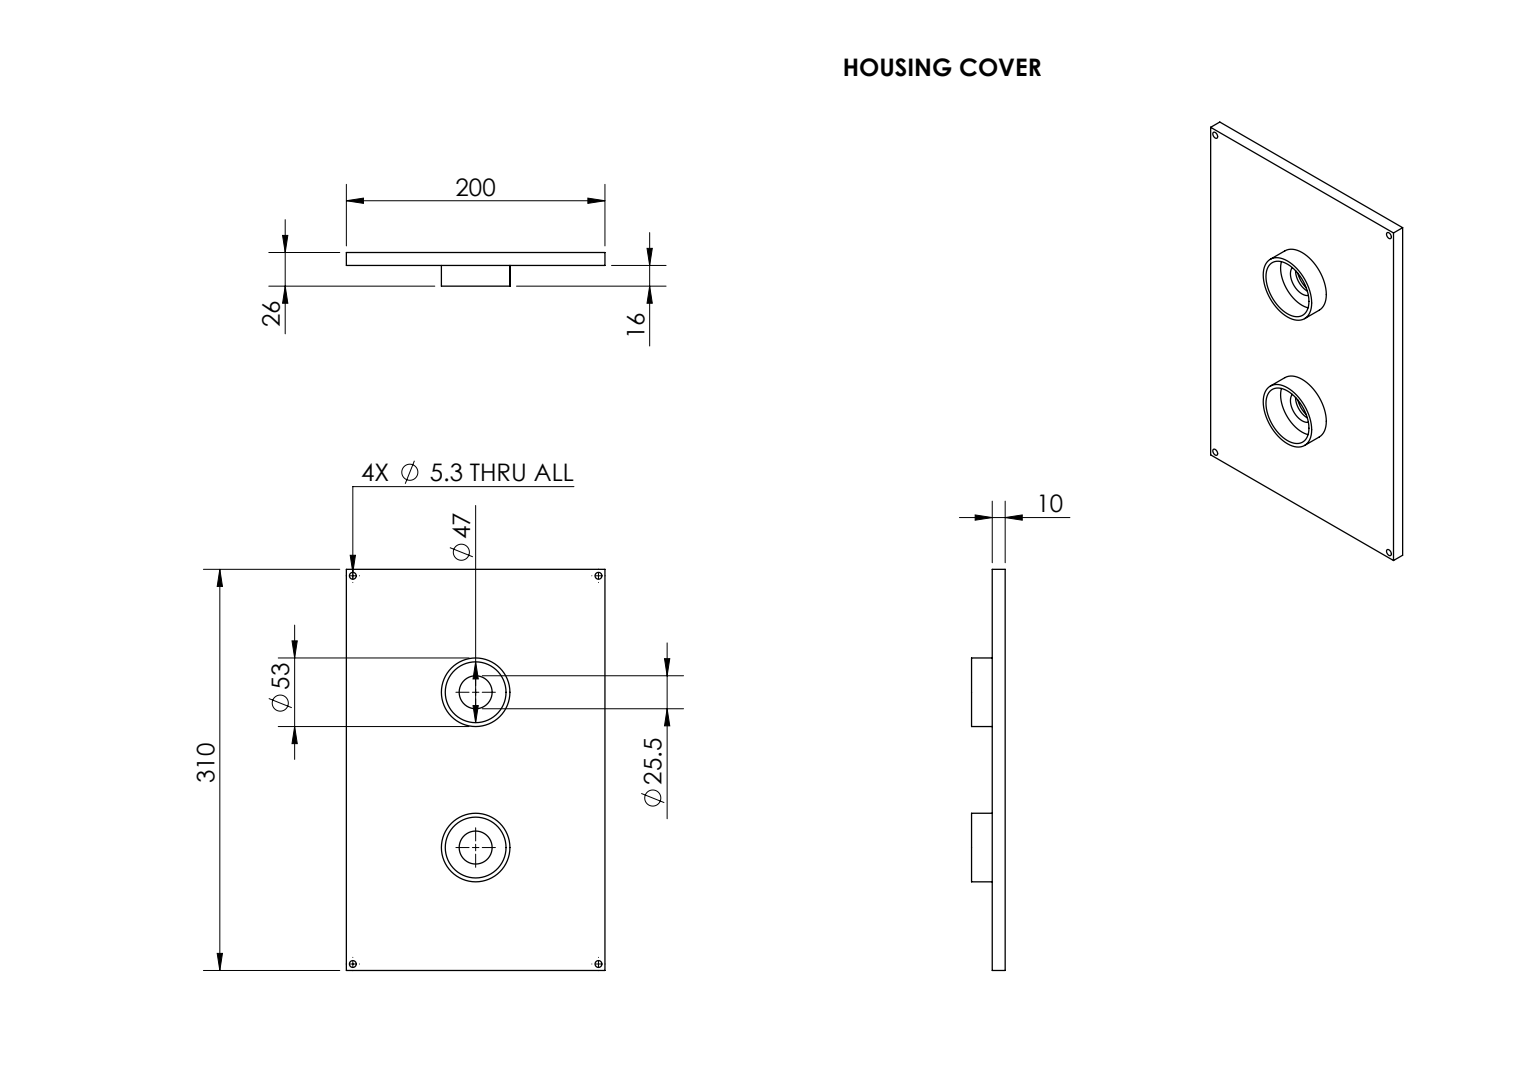
ISO-10303-21;
HEADER;
FILE_DESCRIPTION (('STEP AP214'),
    '1' );
FILE_NAME ('housing cover.step',
    '2026-10-08T09:53:37',
    ( '' ),
    ( '' ),
    'SwSTEP 2.0',
    'SolidWorks 2026',
    '' );
FILE_SCHEMA (( 'AUTOMOTIVE_DESIGN' ));
ENDSEC;

DATA;
#75=VERTEX_POINT ( 'NONE', #9336 ) ;
#149=ORIENTED_EDGE ( 'NONE', *, *, #29009, .F. ) ;
#225=AXIS2_PLACEMENT_3D ( 'NONE', #13248, #59124, #26003 ) ;
#235=EDGE_CURVE ( 'NONE', #35660, #27140, #36937, .T. ) ;
#309=CARTESIAN_POINT ( 'NONE',  ( -100.0000000000260485, 95.00000000000001421, -75.00000000000000000 ) ) ;
#339=DIRECTION ( 'NONE',  ( -1.000000000000000000, 7.571537405616606460E-15, 2.598394312951952234E-14 ) ) ;
#353=ORIENTED_EDGE ( 'NONE', *, *, #72482, .T. ) ;
#452=CYLINDRICAL_SURFACE ( 'NONE', #60264, 2.650000000000540812 ) ;
#531=LINE ( 'NONE', #23425, #23947 ) ;
#665=VECTOR ( 'NONE', #62386, 1000.000000000000000 ) ;
#686=ORIENTED_EDGE ( 'NONE', *, *, #12634, .T. ) ;
#690=CARTESIAN_POINT ( 'NONE',  ( 23.50000000000218847, -119.9999999999999716, -48.99999999999936051 ) ) ;
#767=AXIS2_PLACEMENT_3D ( 'NONE', #73077, #44536, #67455 ) ;
#820=DIRECTION ( 'NONE',  ( -2.603472992746261562E-14, -2.546204323184492723E-14, 1.000000000000000000 ) ) ;
#840=CARTESIAN_POINT ( 'NONE',  ( -0.0004442498512760095037, 0.001194404164628348752, -49.00000000000000000 ) ) ;
#873=LINE ( 'NONE', #58714, #8919 ) ;
#960=ORIENTED_EDGE ( 'NONE', *, *, #66954, .T. ) ;
#1095=VECTOR ( 'NONE', #67288, 1000.000000000000000 ) ;
#1388=DIRECTION ( 'NONE',  ( -1.000000000000000000, 7.955419762439749020E-15, 2.563413034563919251E-14 ) ) ;
#1416=ADVANCED_FACE ( 'NONE', ( #10037 ), #32956, .F. ) ;
#1664=FACE_OUTER_BOUND ( 'NONE', #62733, .T. ) ;
#1775=CIRCLE ( 'NONE', #40207, 12.75000000000265565 ) ;
#1848=CARTESIAN_POINT ( 'NONE',  ( 95.00000000002596323, -209.9999999999999147, -64.99999999999349143 ) ) ;
#1879=CIRCLE ( 'NONE', #16226, 26.50000000000552092 ) ;
#2199=CYLINDRICAL_SURFACE ( 'NONE', #34816, 2.650000000000540812 ) ;
#2442=ADVANCED_FACE ( 'NONE', ( #59711 ), #30006, .F. ) ;
#2449=AXIS2_PLACEMENT_3D ( 'NONE', #19349, #59212, #6604 ) ;
#2456=VERTEX_POINT ( 'NONE', #70970 ) ;
#2468=DIRECTION ( 'NONE',  ( 1.000000000000000000, -7.571539615859142926E-15, -2.592266024478009537E-14 ) ) ;
#2785=CARTESIAN_POINT ( 'NONE',  ( -100.0000000000260485, 95.00000000000001421, 75.00000000000001421 ) ) ;
#2842=ORIENTED_EDGE ( 'NONE', *, *, #51935, .T. ) ;
#2994=ADVANCED_FACE ( 'NONE', ( #23240 ), #21740, .F. ) ;
#3108=PLANE ( 'NONE',  #225 ) ;
#3141=DIRECTION ( 'NONE',  ( 2.603472992746261562E-14, 2.546204323184492723E-14, -1.000000000000000000 ) ) ;
#3340=DIRECTION ( 'NONE',  ( -1.000000000000000000, 7.571543891232750625E-15, 2.563413034563919882E-14 ) ) ;
#3419=VECTOR ( 'NONE', #71589, 1000.000000000000000 ) ;
#3801=FACE_OUTER_BOUND ( 'NONE', #55805, .T. ) ;
#4047=LINE ( 'NONE', #26942, #70051 ) ;
#4203=ORIENTED_EDGE ( 'NONE', *, *, #69812, .T. ) ;
#4207=ADVANCED_FACE ( 'NONE', ( #71116, #8723 ), #3108, .T. ) ;
#4229=DIRECTION ( 'NONE',  ( -1.000000000000000000, 7.677074106448950501E-15, 2.598394312951952234E-14 ) ) ;
#4446=FACE_OUTER_BOUND ( 'NONE', #31443, .T. ) ;
#4524=LINE ( 'NONE', #61285, #1095 ) ;
#4609=AXIS2_PLACEMENT_3D ( 'NONE', #43719, #49336, #66995 ) ;
#4688=CARTESIAN_POINT ( 'NONE',  ( -0.0004442498507136653329, 0.001194404164628348752, -70.59999999999999432 ) ) ;
#4779=VECTOR ( 'NONE', #23199, 1000.000000000000000 ) ;
#4855=CARTESIAN_POINT ( 'NONE',  ( -0.0004442498512760095037, 0.001194404164628348752, -49.00000000000000000 ) ) ;
#4888=DIRECTION ( 'NONE',  ( -1.000000000000000000, 5.236901059551556403E-15, 2.618450529775778123E-14 ) ) ;
#4891=DIRECTION ( 'NONE',  ( -1.000000000000000000, 1.047380211910311281E-14, 2.618450529775778123E-14 ) ) ;
#4973=VECTOR ( 'NONE', #29994, 1000.000000000000000 ) ;
#5079=COLOUR_RGB ( '', 0.66274510, 0.83137255, 0.94901961) ;
#5184=AXIS2_PLACEMENT_3D ( 'NONE', #13484, #8955, #36780 ) ;
#5204=( NAMED_UNIT ( * ) PLANE_ANGLE_UNIT ( ) SI_UNIT ( $, .RADIAN. ) );
#5224=DIRECTION ( 'NONE',  ( -1.000000000000000000, 7.571544473058805744E-15, 2.612289469705706870E-14 ) ) ;
#5225=ORIENTED_EDGE ( 'NONE', *, *, #49422, .T. ) ;
#5233=EDGE_CURVE ( 'NONE', #22100, #20743, #33218, .T. ) ;
#5362=EDGE_CURVE ( 'NONE', #75, #7432, #54715, .T. ) ;
#5427=CARTESIAN_POINT ( 'NONE',  ( -100.0000000000260059, -214.9999999999999716, 75.00000000001300293 ) ) ;
#5570=EDGE_LOOP ( 'NONE', ( #66507, #70540, #51036, #5665 ) ) ;
#5573=LINE ( 'NONE', #39398, #68174 ) ;
#5609=CARTESIAN_POINT ( 'NONE',  ( 1.692257445284848207E-12, 0.000000000000000000, -65.00000000000000000 ) ) ;
#5612=EDGE_CURVE ( 'NONE', #64620, #51781, #64388, .T. ) ;
#5619=DIRECTION ( 'NONE',  ( 2.603472992746261562E-14, 2.546204323184492723E-14, -1.000000000000000000 ) ) ;
#5665=ORIENTED_EDGE ( 'NONE', *, *, #64179, .F. ) ;
#5726=DIRECTION ( 'NONE',  ( 2.603472992746261562E-14, 2.546204323184492723E-14, -1.000000000000000000 ) ) ;
#5837=ORIENTED_EDGE ( 'NONE', *, *, #8050, .F. ) ;
#5860=ORIENTED_EDGE ( 'NONE', *, *, #50226, .F. ) ;
#5883=CYLINDRICAL_SURFACE ( 'NONE', #15596, 2.650000000000540812 ) ;
#5913=AXIS2_PLACEMENT_3D ( 'NONE', #70534, #20538, #66412 ) ;
#5943=SURFACE_STYLE_USAGE ( .BOTH. , #40137 ) ;
#5966=CARTESIAN_POINT ( 'NONE',  ( 95.00000000002596323, -209.9999999999999147, -74.99999999999349143 ) ) ;
#6234=DIRECTION ( 'NONE',  ( -1.000000000000000000, 7.571541139944061634E-15, 2.603472992745718826E-14 ) ) ;
#6399=FACE_OUTER_BOUND ( 'NONE', #37814, .T. ) ;
#6400=EDGE_CURVE ( 'NONE', #46991, #57518, #64592, .T. ) ;
#6460=DIRECTION ( 'NONE',  ( -1.000000000000000000, 1.047380211910311281E-14, 2.618450529775778123E-14 ) ) ;
#6484=EDGE_CURVE ( 'NONE', #55201, #43013, #21999, .T. ) ;
#6562=EDGE_CURVE ( 'NONE', #6768, #30711, #66814, .T. ) ;
#6604=DIRECTION ( 'NONE',  ( 1.000000000000000000, -7.331661483372147883E-15, -2.618450529775767079E-14 ) ) ;
#6633=AXIS2_PLACEMENT_3D ( 'NONE', #30357, #53302, #68759 ) ;
#6748=ORIENTED_EDGE ( 'NONE', *, *, #72073, .T. ) ;
#6768=VERTEX_POINT ( 'NONE', #22819 ) ;
#6798=EDGE_CURVE ( 'NONE', #52133, #14126, #31591, .T. ) ;
#6966=FACE_BOUND ( 'NONE', #58248, .T. ) ;
#7043=ADVANCED_FACE ( 'NONE', ( #9205 ), #20107, .F. ) ;
#7102=( NAMED_UNIT ( * ) SI_UNIT ( $, .STERADIAN. ) SOLID_ANGLE_UNIT ( ) );
#7116=VECTOR ( 'NONE', #65821, 1000.000000000000000 ) ;
#7300=ORIENTED_EDGE ( 'NONE', *, *, #67968, .T. ) ;
#7314=ORIENTED_EDGE ( 'NONE', *, *, #40834, .T. ) ;
#7352=FACE_BOUND ( 'NONE', #46868, .T. ) ;
#7414=EDGE_CURVE ( 'NONE', #49091, #67107, #23299, .T. ) ;
#7432=VERTEX_POINT ( 'NONE', #58557 ) ;
#7636=LINE ( 'NONE', #26027, #7750 ) ;
#7668=DIRECTION ( 'NONE',  ( 2.603472992746261562E-14, 2.546204323184492723E-14, -1.000000000000000000 ) ) ;
#7690=LINE ( 'NONE', #70091, #54295 ) ;
#7703=CIRCLE ( 'NONE', #34100, 2.650000000000540812 ) ;
#7750=VECTOR ( 'NONE', #71142, 1000.000000000000000 ) ;
#7840=ORIENTED_EDGE ( 'NONE', *, *, #5233, .T. ) ;
#7863=EDGE_LOOP ( 'NONE', ( #49210, #51401, #64566, #45309 ) ) ;
#7920=DIRECTION ( 'NONE',  ( 2.603472992746261562E-14, 2.546204323184492723E-14, -1.000000000000000000 ) ) ;
#8001=DIRECTION ( 'NONE',  ( 2.603472992746261562E-14, 2.546204323184492723E-14, -1.000000000000000000 ) ) ;
#8050=EDGE_CURVE ( 'NONE', #22100, #25604, #71592, .T. ) ;
#8245=CIRCLE ( 'NONE', #43094, 15.70000000000326956 ) ;
#8272=DIRECTION ( 'NONE',  ( 1.000000000000000000, 7.705842312278612278E-15, -2.603472992745757322E-14 ) ) ;
#8281=CIRCLE ( 'NONE', #46716, 2.650000000000540812 ) ;
#8322=ORIENTED_EDGE ( 'NONE', *, *, #10250, .T. ) ;
#8346=EDGE_LOOP ( 'NONE', ( #14630, #70144 ) ) ;
#8485=ADVANCED_FACE ( 'NONE', ( #1664, #40738 ), #12883, .T. ) ;
#8538=DIRECTION ( 'NONE',  ( -1.000000000000000000, 7.955419762439749020E-15, 2.563413034563919251E-14 ) ) ;
#8610=CYLINDRICAL_SURFACE ( 'NONE', #37131, 23.50000000000489919 ) ;
#8715=AXIS2_PLACEMENT_3D ( 'NONE', #4688, #74197, #50136 ) ;
#8723=FACE_OUTER_BOUND ( 'NONE', #71462, .T. ) ;
#8892=ORIENTED_EDGE ( 'NONE', *, *, #22702, .F. ) ;
#8901=CARTESIAN_POINT ( 'NONE',  ( 2.861260715122138586E-12, -120.0000000000000000, -75.00000000000000000 ) ) ;
#8906=EDGE_CURVE ( 'NONE', #42522, #22100, #70571, .T. ) ;
#8919=VECTOR ( 'NONE', #64363, 1000.000000000000000 ) ;
#8955=DIRECTION ( 'NONE',  ( -2.603472992746261562E-14, -2.546204323184492723E-14, 1.000000000000000000 ) ) ;
#8981=DIRECTION ( 'NONE',  ( 2.603472992746261562E-14, 2.546204323184492723E-14, -1.000000000000000000 ) ) ;
#9143=PRODUCT_DEFINITION_SHAPE ( 'NONE', 'NONE',  #31551 ) ;
#9205=FACE_OUTER_BOUND ( 'NONE', #18582, .T. ) ;
#9263=DIRECTION ( 'NONE',  ( -2.603472992746261562E-14, -2.546204323184492723E-14, 1.000000000000000000 ) ) ;
#9336=CARTESIAN_POINT ( 'NONE',  ( -92.35000000002612808, 89.99999999999992895, -74.99999999999992895 ) ) ;
#9493=DIRECTION ( 'NONE',  ( 2.603472992746261562E-14, 2.546204323184492723E-14, -1.000000000000000000 ) ) ;
#9614=EDGE_CURVE ( 'NONE', #64620, #52133, #33989, .T. ) ;
#9626=LINE ( 'NONE', #67136, #51555 ) ;
#9698=DIRECTION ( 'NONE',  ( 2.603472992746261562E-14, 2.546204323184492723E-14, -1.000000000000000000 ) ) ;
#9849=CYLINDRICAL_SURFACE ( 'NONE', #24494, 23.50000000000489919 ) ;
#9867=ORIENTED_EDGE ( 'NONE', *, *, #51725, .T. ) ;
#9970=DIRECTION ( 'NONE',  ( 2.603472992746261562E-14, 2.546204323184492723E-14, -1.000000000000000000 ) ) ;
#9980=ORIENTED_EDGE ( 'NONE', *, *, #42054, .T. ) ;
#10036=AXIS2_PLACEMENT_3D ( 'NONE', #43811, #31757, #55442 ) ;
#10037=FACE_OUTER_BOUND ( 'NONE', #23609, .T. ) ;
#10227=DIRECTION ( 'NONE',  ( -7.571541139946887334E-15, 1.000000000000000000, 2.546204323184473159E-14 ) ) ;
#10250=EDGE_CURVE ( 'NONE', #25604, #73822, #39518, .T. ) ;
#10297=DIRECTION ( 'NONE',  ( 2.603472992745699578E-14, -2.546204323184531851E-14, 1.000000000000000000 ) ) ;
#10346=CYLINDRICAL_SURFACE ( 'NONE', #53211, 12.75000000000265565 ) ;
#10395=VERTEX_POINT ( 'NONE', #19525 ) ;
#10400=MECHANICAL_DESIGN_GEOMETRIC_PRESENTATION_REPRESENTATION('',(#28426),#23610);
#10430=DIRECTION ( 'NONE',  ( -1.000000000000000000, 7.571539615859142926E-15, 2.592266024478009537E-14 ) ) ;
#10480=FACE_BOUND ( 'NONE', #35331, .T. ) ;
#10514=FILL_AREA_STYLE_COLOUR ( '', #18810 ) ;
#10593=CARTESIAN_POINT ( 'NONE',  ( 2.746707903440850533E-12, -120.0000000000000000, -70.59999999999999432 ) ) ;
#10809=CIRCLE ( 'NONE', #45664, 12.75000000000265565 ) ;
#10887=CARTESIAN_POINT ( 'NONE',  ( -15.70044424985387188, 0.001194404164747221980, -74.99999999999958789 ) ) ;
#10892=ADVANCED_FACE ( 'NONE', ( #42388 ), #2199, .F. ) ;
#11106=DIRECTION ( 'NONE',  ( 2.603472992746261562E-14, 2.546204323184492723E-14, -1.000000000000000000 ) ) ;
#11125=ADVANCED_FACE ( 'NONE', ( #66075 ), #5883, .F. ) ;
#11158=CARTESIAN_POINT ( 'NONE',  ( 26.49955575014914189, 0.001194404164634644498, -64.99999999999930367 ) ) ;
#11179=CARTESIAN_POINT ( 'NONE',  ( -0.0004442498512760095037, 0.001194404164628348752, -49.00000000000000000 ) ) ;
#11423=DIRECTION ( 'NONE',  ( 2.603472992746261562E-14, 2.546204323184492723E-14, -1.000000000000000000 ) ) ;
#11448=ORIENTED_EDGE ( 'NONE', *, *, #19451, .T. ) ;
#11479=ORIENTED_EDGE ( 'NONE', *, *, #70861, .T. ) ;
#11501=DIRECTION ( 'NONE',  ( 2.603472992746261562E-14, 2.546204323184492723E-14, -1.000000000000000000 ) ) ;
#11616=ORIENTED_EDGE ( 'NONE', *, *, #63442, .T. ) ;
#11629=ORIENTED_EDGE ( 'NONE', *, *, #46112, .T. ) ;
#11782=CIRCLE ( 'NONE', #34598, 15.70000000000326956 ) ;
#11845=ADVANCED_FACE ( 'NONE', ( #67637 ), #66530, .F. ) ;
#11937=ORIENTED_EDGE ( 'NONE', *, *, #9614, .F. ) ;
#12024=VECTOR ( 'NONE', #59259, 1000.000000000000000 ) ;
#12175=FACE_OUTER_BOUND ( 'NONE', #28138, .T. ) ;
#12199=ORIENTED_EDGE ( 'NONE', *, *, #45524, .T. ) ;
#12209=CARTESIAN_POINT ( 'NONE',  ( 23.50000000000260414, -119.9999999999999716, -64.99999999999938893 ) ) ;
#12296=DIRECTION ( 'NONE',  ( 2.603472992746261562E-14, 2.546204323184492723E-14, -1.000000000000000000 ) ) ;
#12317=CIRCLE ( 'NONE', #53159, 2.650000000000540812 ) ;
#12387=AXIS2_PLACEMENT_3D ( 'NONE', #1848, #48405, #30366 ) ;
#12417=VECTOR ( 'NONE', #64516, 1000.000000000000000 ) ;
#12534=DIRECTION ( 'NONE',  ( -1.000000000000000000, 7.677074106448950501E-15, 2.598394312951952234E-14 ) ) ;
#12627=LINE ( 'NONE', #35565, #12417 ) ;
#12634=EDGE_CURVE ( 'NONE', #10395, #2456, #65815, .T. ) ;
#12779=EDGE_LOOP ( 'NONE', ( #43223, #52931, #15236, #53707 ) ) ;
#12814=VECTOR ( 'NONE', #59888, 1000.000000000000000 ) ;
#12841=VECTOR ( 'NONE', #37141, 1000.000000000000000 ) ;
#12883=PLANE ( 'NONE',  #66193 ) ;
#12972=ORIENTED_EDGE ( 'NONE', *, *, #23448, .F. ) ;
#13036=ORIENTED_EDGE ( 'NONE', *, *, #8906, .T. ) ;
#13180=CIRCLE ( 'NONE', #2449, 26.50000000000552092 ) ;
#13248=CARTESIAN_POINT ( 'NONE',  ( 1.692257445284848207E-12, 0.000000000000000000, -65.00000000000000000 ) ) ;
#13256=ORIENTED_EDGE ( 'NONE', *, *, #50505, .T. ) ;
#13284=DIRECTION ( 'NONE',  ( 2.603472992746261562E-14, 2.546204323184492723E-14, -1.000000000000000000 ) ) ;
#13431=VECTOR ( 'NONE', #37597, 1000.000000000000000 ) ;
#13451=CARTESIAN_POINT ( 'NONE',  ( -100.0000000000260485, 95.00000000000001421, -65.00000000000001421 ) ) ;
#13484=CARTESIAN_POINT ( 'NONE',  ( -95.00000000002611955, 90.00000000000007105, -65.00000000000000000 ) ) ;
#13501=CARTESIAN_POINT ( 'NONE',  ( 15.70000000000286455, -120.0000000000000568, -74.99999999999958789 ) ) ;
#13580=EDGE_CURVE ( 'NONE', #7432, #75, #39527, .T. ) ;
#13870=ORIENTED_EDGE ( 'NONE', *, *, #41853, .F. ) ;
#13932=ADVANCED_BREP_SHAPE_REPRESENTATION ( '', ( #38137, #43395 ), #37485 ) ;
#13942=CARTESIAN_POINT ( 'NONE',  ( 97.65000000002596892, 89.99999999999992895, -74.99999999999992895 ) ) ;
#13989=DIRECTION ( 'NONE',  ( 1.000000000000000000, -5.236901059551556403E-15, -2.618450529775778123E-14 ) ) ;
#14031=VERTEX_POINT ( 'NONE', #14326 ) ;
#14126=VERTEX_POINT ( 'NONE', #13942 ) ;
#14235=EDGE_LOOP ( 'NONE', ( #57149, #9867 ) ) ;
#14296=DIRECTION ( 'NONE',  ( 2.603472992746261562E-14, 2.546204323184492723E-14, -1.000000000000000000 ) ) ;
#14326=CARTESIAN_POINT ( 'NONE',  ( 26.50000000000260414, -120.0000000000000000, -64.99999999999930367 ) ) ;
#14362=CARTESIAN_POINT ( 'NONE',  ( -23.50044424985086522, 0.001194404165009976208, -65.00000000000061107 ) ) ;
#14441=EDGE_LOOP ( 'NONE', ( #68414, #686, #11629, #48567 ) ) ;
#14484=CARTESIAN_POINT ( 'NONE',  ( 12.74955575014928399, 0.001194404169505926478, -70.59999999999966747 ) ) ;
#14630=ORIENTED_EDGE ( 'NONE', *, *, #48541, .F. ) ;
#14786=ORIENTED_EDGE ( 'NONE', *, *, #41200, .F. ) ;
#14904=CARTESIAN_POINT ( 'NONE',  ( 2.184357737007946383E-12, -120.0000000000000000, -48.99999999999997158 ) ) ;
#14961=EDGE_LOOP ( 'NONE', ( #17025, #62430, #44757, #58599 ) ) ;
#15035=CARTESIAN_POINT ( 'NONE',  ( -12.75000000000506617, -119.9999999999999005, 127.5000000000003411 ) ) ;
#15051=VERTEX_POINT ( 'NONE', #16019 ) ;
#15198=CARTESIAN_POINT ( 'NONE',  ( 2.184357737007946383E-12, -120.0000000000000000, -48.99999999999997158 ) ) ;
#15236=ORIENTED_EDGE ( 'NONE', *, *, #41200, .T. ) ;
#15262=DIRECTION ( 'NONE',  ( 1.000000000000000000, -7.677074106448950501E-15, -2.598394312951952234E-14 ) ) ;
#15324=CARTESIAN_POINT ( 'NONE',  ( 2.746707903440850533E-12, -120.0000000000000000, -70.59999999999999432 ) ) ;
#15378=CARTESIAN_POINT ( 'NONE',  ( -95.00000000002617639, -209.9999999999999432, -74.99999999999349143 ) ) ;
#15468=ORIENTED_EDGE ( 'NONE', *, *, #71520, .T. ) ;
#15550=CARTESIAN_POINT ( 'NONE',  ( 92.35000000002543175, -209.9999999999998863, -74.99999999999342037 ) ) ;
#15583=CARTESIAN_POINT ( 'NONE',  ( 2.746707903440850533E-12, -120.0000000000000000, -70.59999999999999432 ) ) ;
#15596=AXIS2_PLACEMENT_3D ( 'NONE', #67912, #63037, #56643 ) ;
#15630=ORIENTED_EDGE ( 'NONE', *, *, #44237, .T. ) ;
#15684=DIRECTION ( 'NONE',  ( 2.603472992746261562E-14, 2.546204323184492723E-14, -1.000000000000000000 ) ) ;
#15864=FACE_OUTER_BOUND ( 'NONE', #14961, .T. ) ;
#15882=ADVANCED_FACE ( 'NONE', ( #50183 ), #10346, .F. ) ;
#15906=EDGE_LOOP ( 'NONE', ( #37945, #70321, #33393, #47519 ) ) ;
#15970=ORIENTED_EDGE ( 'NONE', *, *, #51700, .T. ) ;
#16019=CARTESIAN_POINT ( 'NONE',  ( 15.69955575014939875, 0.001194404164567414856, -74.99999999999958789 ) ) ;
#16226=AXIS2_PLACEMENT_3D ( 'NONE', #14904, #9263, #66779 ) ;
#16499=DIRECTION ( 'NONE',  ( 1.000000000000000000, -7.571541139944063212E-15, -2.603472992745718826E-14 ) ) ;
#16509=CYLINDRICAL_SURFACE ( 'NONE', #62344, 26.50000000000552092 ) ;
#16541=DIRECTION ( 'NONE',  ( 2.603472992745699578E-14, -2.546204323184531851E-14, 1.000000000000000000 ) ) ;
#16692=FACE_BOUND ( 'NONE', #51137, .T. ) ;
#16699=PLANE ( 'NONE',  #67969 ) ;
#17025=ORIENTED_EDGE ( 'NONE', *, *, #72948, .T. ) ;
#17085=DIRECTION ( 'NONE',  ( -2.603472992746261562E-14, -2.546204323184492723E-14, 1.000000000000000000 ) ) ;
#17145=VERTEX_POINT ( 'NONE', #48728 ) ;
#17206=SURFACE_STYLE_FILL_AREA ( #22859 ) ;
#17222=CARTESIAN_POINT ( 'NONE',  ( 15.70000000000274909, -120.0000000000000568, -70.59999999999959641 ) ) ;
#17330=FACE_OUTER_BOUND ( 'NONE', #66485, .T. ) ;
#17356=DIRECTION ( 'NONE',  ( -2.603472992746261562E-14, -2.546204323184492723E-14, 1.000000000000000000 ) ) ;
#17366=CIRCLE ( 'NONE', #59394, 12.75000000000265388 ) ;
#17371=LINE ( 'NONE', #40303, #22485 ) ;
#17430=CARTESIAN_POINT ( 'NONE',  ( 95.00000000002596323, -209.9999999999999147, -64.99999999999349143 ) ) ;
#17462=CARTESIAN_POINT ( 'NONE',  ( -0.0004442498505991059293, 0.001194404164628348752, -75.00000000000000000 ) ) ;
#17492=VERTEX_POINT ( 'NONE', #12209 ) ;
#17537=DIRECTION ( 'NONE',  ( 2.603472992746261562E-14, 2.546204323184492723E-14, -1.000000000000000000 ) ) ;
#17597=AXIS2_PLACEMENT_3D ( 'NONE', #36040, #34940, #58986 ) ;
#17666=PLANE ( 'NONE',  #63430 ) ;
#17865=AXIS2_PLACEMENT_3D ( 'NONE', #61847, #27627, #33250 ) ;
#17885=AXIS2_PLACEMENT_3D ( 'NONE', #31330, #7668, #60663 ) ;
#17908=CARTESIAN_POINT ( 'NONE',  ( 2.600855584879231068E-12, -120.0000000000000000, -65.00000000000000000 ) ) ;
#17973=DIRECTION ( 'NONE',  ( -2.603472992746261562E-14, -2.546204323184492723E-14, 1.000000000000000000 ) ) ;
#17991=CARTESIAN_POINT ( 'NONE',  ( 2.184357737007946383E-12, -120.0000000000000000, -48.99999999999997158 ) ) ;
#18031=FACE_BOUND ( 'NONE', #35522, .T. ) ;
#18145=ORIENTED_EDGE ( 'NONE', *, *, #67148, .F. ) ;
#18161=VERTEX_POINT ( 'NONE', #28123 ) ;
#18206=VERTEX_POINT ( 'NONE', #17222 ) ;
#18334=CARTESIAN_POINT ( 'NONE',  ( -95.00000000002617639, -209.9999999999999432, -74.99999999999349143 ) ) ;
#18373=( LENGTH_UNIT ( ) NAMED_UNIT ( * ) SI_UNIT ( .MILLI., .METRE. ) );
#18416=ORIENTED_EDGE ( 'NONE', *, *, #70585, .T. ) ;
#18492=ORIENTED_EDGE ( 'NONE', *, *, #50859, .T. ) ;
#18554=CARTESIAN_POINT ( 'NONE',  ( 95.00000000002597744, 90.00000000000007105, -75.00000000000000000 ) ) ;
#18582=EDGE_LOOP ( 'NONE', ( #38224, #8322, #960, #31703 ) ) ;
#18635=EDGE_LOOP ( 'NONE', ( #29830, #23329, #68263, #7300 ) ) ;
#18739=AXIS2_PLACEMENT_3D ( 'NONE', #15583, #61076, #55434 ) ;
#18741=( NAMED_UNIT ( * ) PLANE_ANGLE_UNIT ( ) SI_UNIT ( $, .RADIAN. ) );
#18810=COLOUR_RGB ( '', 0.66274510, 0.83137255, 0.94901961) ;
#18954=CIRCLE ( 'NONE', #35744, 12.75000000000265388 ) ;
#18972=ORIENTED_EDGE ( 'NONE', *, *, #70318, .T. ) ;
#19004=ORIENTED_EDGE ( 'NONE', *, *, #52973, .T. ) ;
#19079=CIRCLE ( 'NONE', #5913, 2.650000000000540812 ) ;
#19101=CARTESIAN_POINT ( 'NONE',  ( 100.0000000000260201, 95.00000000000001421, -75.00000000000000000 ) ) ;
#19269=CARTESIAN_POINT ( 'NONE',  ( -100.0000000000260059, -214.9999999999999716, -64.99999999999350564 ) ) ;
#19280=AXIS2_PLACEMENT_3D ( 'NONE', #8901, #53651, #8538 ) ;
#19349=CARTESIAN_POINT ( 'NONE',  ( 2.600913415846943225E-12, -120.0000000000000000, -65.00000000000000000 ) ) ;
#19451=EDGE_CURVE ( 'NONE', #46991, #35660, #17366, .T. ) ;
#19525=CARTESIAN_POINT ( 'NONE',  ( -92.35000000002612808, 89.99999999999992895, -64.99999999999992895 ) ) ;
#19641=DIRECTION ( 'NONE',  ( 1.000000000000000000, -7.677074106448950501E-15, -2.598394312951952234E-14 ) ) ;
#19688=ORIENTED_EDGE ( 'NONE', *, *, #22702, .T. ) ;
#19735=DIRECTION ( 'NONE',  ( 1.000000000000000000, 0.000000000000000000, 0.000000000000000000 ) ) ;
#19841=EDGE_CURVE ( 'NONE', #51781, #64620, #73817, .T. ) ;
#19942=ORIENTED_EDGE ( 'NONE', *, *, #6400, .F. ) ;
#19946=ORIENTED_EDGE ( 'NONE', *, *, #60446, .T. ) ;
#20094=DIRECTION ( 'NONE',  ( 1.000000000000000000, -7.571541139944061634E-15, -2.603472992745718826E-14 ) ) ;
#20107=PLANE ( 'NONE',  #10036 ) ;
#20153=AXIS2_PLACEMENT_3D ( 'NONE', #24557, #8001, #70392 ) ;
#20295=UNCERTAINTY_MEASURE_WITH_UNIT (LENGTH_MEASURE( 1.000000000000000082E-05 ), #44678, 'distance_accuracy_value', 'NONE');
#20306=LINE ( 'NONE', #21039, #67116 ) ;
#20361=CARTESIAN_POINT ( 'NONE',  ( -92.35000000002563070, -209.9999999999999716, -74.99999999999356248 ) ) ;
#20477=LINE ( 'NONE', #25741, #3419 ) ;
#20538=DIRECTION ( 'NONE',  ( -2.603472992746261562E-14, -2.546204323184492723E-14, 1.000000000000000000 ) ) ;
#20743=VERTEX_POINT ( 'NONE', #73895 ) ;
#20811=DIRECTION ( 'NONE',  ( 1.000000000000000000, -5.236901059551556403E-15, -2.618450529775778123E-14 ) ) ;
#20840=CARTESIAN_POINT ( 'NONE',  ( 2.600913415846943225E-12, -120.0000000000000000, -65.00000000000000000 ) ) ;
#20860=CARTESIAN_POINT ( 'NONE',  ( 97.65000000002596892, 89.99999999999992895, -64.99999999999992895 ) ) ;
#20885=AXIS2_PLACEMENT_3D ( 'NONE', #33240, #17085, #51284 ) ;
#20924=AXIS2_PLACEMENT_3D ( 'NONE', #35997, #17973, #64217 ) ;
#21002=CIRCLE ( 'NONE', #6633, 12.75000000000265388 ) ;
#21039=CARTESIAN_POINT ( 'NONE',  ( 23.49955575015362186, 0.001194404164453295421, -49.00000000000061107 ) ) ;
#21365=ORIENTED_EDGE ( 'NONE', *, *, #52973, .F. ) ;
#21375=CARTESIAN_POINT ( 'NONE',  ( 100.0000000000260201, 95.00000000000001421, -75.00000000000000000 ) ) ;
#21517=VERTEX_POINT ( 'NONE', #34521 ) ;
#21616=ORIENTED_EDGE ( 'NONE', *, *, #42890, .F. ) ;
#21692=VECTOR ( 'NONE', #20094, 1000.000000000000000 ) ;
#21710=ORIENTED_EDGE ( 'NONE', *, *, #69910, .F. ) ;
#21740=CYLINDRICAL_SURFACE ( 'NONE', #22586, 23.50000000000489919 ) ;
#21796=ADVANCED_FACE ( 'NONE', ( #67448, #34343, #32850, #16692, #27201, #38880, #45653 ), #61820, .F. ) ;
#21821=EDGE_CURVE ( 'NONE', #35409, #63658, #31501, .T. ) ;
#21873=CARTESIAN_POINT ( 'NONE',  ( 15.69955575015255533, 0.001194404164511398249, -70.60000000000039222 ) ) ;
#21999=CIRCLE ( 'NONE', #12387, 2.650000000000540812 ) ;
#22015=CARTESIAN_POINT ( 'NONE',  ( -12.74999999999739941, -119.9999999999949267, -65.00000000000034106 ) ) ;
#22100=VERTEX_POINT ( 'NONE', #19269 ) ;
#22177=ORIENTED_EDGE ( 'NONE', *, *, #67148, .T. ) ;
#22179=SURFACE_SIDE_STYLE ('',( #56404 ) ) ;
#22230=CARTESIAN_POINT ( 'NONE',  ( -0.0004442498508594591917, 0.001194404164628348752, -65.00000000000000000 ) ) ;
#22307=ORIENTED_EDGE ( 'NONE', *, *, #46008, .T. ) ;
#22308=AXIS2_PLACEMENT_3D ( 'NONE', #35090, #47479, #59135 ) ;
#22485=VECTOR ( 'NONE', #45594, 1000.000000000000000 ) ;
#22500=DIRECTION ( 'NONE',  ( 2.603472992746261562E-14, 2.546204323184492723E-14, -1.000000000000000000 ) ) ;
#22518=FACE_OUTER_BOUND ( 'NONE', #50874, .T. ) ;
#22553=CARTESIAN_POINT ( 'NONE',  ( -0.0004442498508594591917, 0.001194404164628348752, -65.00000000000000000 ) ) ;
#22561=ORIENTED_EDGE ( 'NONE', *, *, #6798, .F. ) ;
#22573=FACE_BOUND ( 'NONE', #22994, .T. ) ;
#22586=AXIS2_PLACEMENT_3D ( 'NONE', #4855, #67984, #66229 ) ;
#22702=EDGE_CURVE ( 'NONE', #61695, #20743, #25930, .T. ) ;
#22819=CARTESIAN_POINT ( 'NONE',  ( 100.0000000000260201, 95.00000000000001421, -65.00000000000001421 ) ) ;
#22839=CIRCLE ( 'NONE', #64865, 2.650000000000540812 ) ;
#22859=FILL_AREA_STYLE ('',( #65276 ) ) ;
#22955=DIRECTION ( 'NONE',  ( -2.603472992745699578E-14, 2.546204323184531851E-14, -1.000000000000000000 ) ) ;
#22972=AXIS2_PLACEMENT_3D ( 'NONE', #35288, #46569, #69498 ) ;
#22994=EDGE_LOOP ( 'NONE', ( #18145, #32910 ) ) ;
#23035=ORIENTED_EDGE ( 'NONE', *, *, #60584, .F. ) ;
#23132=DIRECTION ( 'NONE',  ( 2.603472992746261562E-14, 2.546204323184492723E-14, -1.000000000000000000 ) ) ;
#23199=DIRECTION ( 'NONE',  ( -1.000000000000000000, 7.571541139944061634E-15, 2.603472992745718826E-14 ) ) ;
#23240=FACE_OUTER_BOUND ( 'NONE', #39583, .T. ) ;
#23292=EDGE_CURVE ( 'NONE', #63726, #18161, #25552, .T. ) ;
#23299=CIRCLE ( 'NONE', #20924, 23.50000000000489919 ) ;
#23329=ORIENTED_EDGE ( 'NONE', *, *, #30205, .F. ) ;
#23425=CARTESIAN_POINT ( 'NONE',  ( 92.35000000002543175, -209.9999999999998863, -74.99999999999342037 ) ) ;
#23448=EDGE_CURVE ( 'NONE', #29601, #31522, #45688, .T. ) ;
#23477=DIRECTION ( 'NONE',  ( -1.000000000000000000, 7.571543891232750625E-15, 2.563413034563919882E-14 ) ) ;
#23609=EDGE_LOOP ( 'NONE', ( #5860, #22307, #11479, #54895 ) ) ;
#23610=( GEOMETRIC_REPRESENTATION_CONTEXT ( 3 ) GLOBAL_UNCERTAINTY_ASSIGNED_CONTEXT ( ( #36844 ) ) GLOBAL_UNIT_ASSIGNED_CONTEXT ( ( #18373, #18741, #7102 ) ) REPRESENTATION_CONTEXT ( 'NONE', 'WORKASPACE' ) );
#23632=CARTESIAN_POINT ( 'NONE',  ( -95.00000000002611955, 90.00000000000007105, -75.00000000000000000 ) ) ;
#23639=CYLINDRICAL_SURFACE ( 'NONE', #22972, 12.75000000000265388 ) ;
#23723=DIRECTION ( 'NONE',  ( 1.000000000000000000, -7.571539615859142926E-15, -2.592266024478009537E-14 ) ) ;
#23735=AXIS2_PLACEMENT_3D ( 'NONE', #29353, #47403, #63227 ) ;
#23871=CARTESIAN_POINT ( 'NONE',  ( 26.50000000000218847, -120.0000000000000000, -48.99999999999928946 ) ) ;
#23932=EDGE_CURVE ( 'NONE', #2456, #10395, #41224, .T. ) ;
#23947=VECTOR ( 'NONE', #46357, 1000.000000000000000 ) ;
#24039=SURFACE_STYLE_USAGE ( .BOTH. , #22179 ) ;
#24121=CYLINDRICAL_SURFACE ( 'NONE', #68984, 2.650000000000540812 ) ;
#24145=ORIENTED_EDGE ( 'NONE', *, *, #72482, .F. ) ;
#24218=ADVANCED_FACE ( 'NONE', ( #4446 ), #66841, .F. ) ;
#24259=EDGE_LOOP ( 'NONE', ( #73975, #54793 ) ) ;
#24494=AXIS2_PLACEMENT_3D ( 'NONE', #72610, #55712, #4229 ) ;
#24557=CARTESIAN_POINT ( 'NONE',  ( -95.00000000002617639, -209.9999999999999432, -74.99999999999349143 ) ) ;
#24594=CARTESIAN_POINT ( 'NONE',  ( -0.0004442498512760095037, 0.001194404164628348752, -49.00000000000000000 ) ) ;
#24639=EDGE_CURVE ( 'NONE', #51781, #14126, #873, .T. ) ;
#24758=ORIENTED_EDGE ( 'NONE', *, *, #70284, .T. ) ;
#24862=VECTOR ( 'NONE', #56065, 1000.000000000000000 ) ;
#24920=DIRECTION ( 'NONE',  ( -2.603472992746261562E-14, -2.546204323184492723E-14, 1.000000000000000000 ) ) ;
#24942=CIRCLE ( 'NONE', #70535, 23.50000000000489919 ) ;
#24945=AXIS2_PLACEMENT_3D ( 'NONE', #10593, #39555, #33149 ) ;
#25033=ORIENTED_EDGE ( 'NONE', *, *, #24639, .F. ) ;
#25042=LINE ( 'NONE', #31419, #12024 ) ;
#25123=CARTESIAN_POINT ( 'NONE',  ( -2.410829926157000802E-12, -120.0000000000000000, 127.5000000000000000 ) ) ;
#25191=VECTOR ( 'NONE', #9493, 1000.000000000000000 ) ;
#25485=EDGE_CURVE ( 'NONE', #31522, #37710, #1775, .T. ) ;
#25508=ORIENTED_EDGE ( 'NONE', *, *, #21821, .F. ) ;
#25509=CIRCLE ( 'NONE', #29159, 23.50000000000489919 ) ;
#25518=ORIENTED_EDGE ( 'NONE', *, *, #19841, .T. ) ;
#25552=CIRCLE ( 'NONE', #54374, 26.50000000000552092 ) ;
#25604=VERTEX_POINT ( 'NONE', #48363 ) ;
#25645=CARTESIAN_POINT ( 'NONE',  ( -95.00000000002617639, -209.9999999999999432, -64.99999999999349143 ) ) ;
#25741=CARTESIAN_POINT ( 'NONE',  ( -26.50000000000333600, -119.9999999999998010, -48.99999999999928946 ) ) ;
#25791=ORIENTED_EDGE ( 'NONE', *, *, #25485, .F. ) ;
#25793=ORIENTED_EDGE ( 'NONE', *, *, #19841, .F. ) ;
#25904=VERTEX_POINT ( 'NONE', #23871 ) ;
#25930=LINE ( 'NONE', #48858, #13431 ) ;
#26003=DIRECTION ( 'NONE',  ( 1.000000000000000000, -7.571541139944063212E-15, -2.603472992745718826E-14 ) ) ;
#26027=CARTESIAN_POINT ( 'NONE',  ( -100.0000000000260059, -214.9999999999999716, -74.99999999999349143 ) ) ;
#26133=EDGE_LOOP ( 'NONE', ( #28478, #25508, #55373, #29321 ) ) ;
#26495=DIRECTION ( 'NONE',  ( -1.000000000000000000, 5.236901059551556403E-15, 2.618450529775778123E-14 ) ) ;
#26638=ORIENTED_EDGE ( 'NONE', *, *, #51367, .F. ) ;
#26791=AXIS2_PLACEMENT_3D ( 'NONE', #23632, #5619, #4888 ) ;
#26848=DIRECTION ( 'NONE',  ( 1.000000000000000000, -7.677074106448950501E-15, -2.598394312951952234E-14 ) ) ;
#26942=CARTESIAN_POINT ( 'NONE',  ( 23.50000000000708411, -120.0000000000001705, -49.00000000000058265 ) ) ;
#27140=VERTEX_POINT ( 'NONE', #70374 ) ;
#27201=FACE_BOUND ( 'NONE', #61304, .T. ) ;
#27212=CARTESIAN_POINT ( 'NONE',  ( -100.0000000000260485, 95.00000000000001421, -65.00000000000001421 ) ) ;
#27260=EDGE_CURVE ( 'NONE', #18206, #40286, #62087, .T. ) ;
#27273=ORIENTED_EDGE ( 'NONE', *, *, #5233, .F. ) ;
#27345=DIRECTION ( 'NONE',  ( -1.000000000000000000, 7.955419762439749020E-15, 2.563413034563919251E-14 ) ) ;
#27368=ORIENTED_EDGE ( 'NONE', *, *, #55071, .T. ) ;
#27469=EDGE_LOOP ( 'NONE', ( #23035, #69582, #34581, #19946 ) ) ;
#27526=CARTESIAN_POINT ( 'NONE',  ( -12.74999999999990941, -119.9999999999999005, -70.59999999999966747 ) ) ;
#27535=ORIENTED_EDGE ( 'NONE', *, *, #5362, .T. ) ;
#27586=PLANE ( 'NONE',  #32266 ) ;
#27593=DIRECTION ( 'NONE',  ( 2.603472992745699578E-14, -2.546204323184531851E-14, 1.000000000000000000 ) ) ;
#27627=DIRECTION ( 'NONE',  ( 2.603472992746261562E-14, 2.546204323184492723E-14, -1.000000000000000000 ) ) ;
#27633=VERTEX_POINT ( 'NONE', #31185 ) ;
#27895=ADVANCED_FACE ( 'NONE', ( #68005, #10480, #6966, #7352, #47199, #33789, #22518 ), #56362, .T. ) ;
#28110=ORIENTED_EDGE ( 'NONE', *, *, #53661, .T. ) ;
#28113=EDGE_CURVE ( 'NONE', #54110, #44982, #20477, .T. ) ;
#28123=CARTESIAN_POINT ( 'NONE',  ( -26.50044424985128089, 0.001194404165032690894, -49.00000000000068923 ) ) ;
#28138=EDGE_LOOP ( 'NONE', ( #28238, #71644, #13256, #11937 ) ) ;
#28238=ORIENTED_EDGE ( 'NONE', *, *, #5612, .T. ) ;
#28275=ORIENTED_EDGE ( 'NONE', *, *, #6484, .T. ) ;
#28324=CARTESIAN_POINT ( 'NONE',  ( 1.952604744559289694E-12, 0.000000000000000000, -75.00000000000000000 ) ) ;
#28426=STYLED_ITEM ( 'NONE', ( #30391 ), #38137 ) ;
#28476=DIRECTION ( 'NONE',  ( 2.603472992746261562E-14, 2.546204323184492723E-14, -1.000000000000000000 ) ) ;
#28478=ORIENTED_EDGE ( 'NONE', *, *, #69812, .F. ) ;
#28527=DIRECTION ( 'NONE',  ( -1.000000000000000000, 1.047380211910311281E-14, 2.618450529775778123E-14 ) ) ;
#28628=DIRECTION ( 'NONE',  ( 2.603472992746261562E-14, 2.546204323184492723E-14, -1.000000000000000000 ) ) ;
#28664=PRODUCT_CONTEXT ( 'NONE', #60386, 'mechanical' ) ;
#28670=CIRCLE ( 'NONE', #74300, 15.70000000000327312 ) ;
#28683=LINE ( 'NONE', #63291, #66777 ) ;
#28852=PRESENTATION_STYLE_ASSIGNMENT (( #5943 ) ) ;
#28965=DIRECTION ( 'NONE',  ( 2.603472992746261562E-14, 2.546204323184492723E-14, -1.000000000000000000 ) ) ;
#28976=DIRECTION ( 'NONE',  ( 2.603472992746261562E-14, 2.546204323184492723E-14, -1.000000000000000000 ) ) ;
#29009=EDGE_CURVE ( 'NONE', #64475, #56506, #8281, .T. ) ;
#29055=EDGE_LOOP ( 'NONE', ( #44842, #71627 ) ) ;
#29122=ADVANCED_FACE ( 'NONE', ( #46205 ), #16509, .T. ) ;
#29159=AXIS2_PLACEMENT_3D ( 'NONE', #20840, #43795, #26848 ) ;
#29196=CIRCLE ( 'NONE', #73641, 12.75000000000265565 ) ;
#29215=EDGE_LOOP ( 'NONE', ( #42575, #45771 ) ) ;
#29321=ORIENTED_EDGE ( 'NONE', *, *, #32420, .T. ) ;
#29325=CARTESIAN_POINT ( 'NONE',  ( 26.49955575014872622, 0.001194404164634644498, -48.99999999999931788 ) ) ;
#29334=CARTESIAN_POINT ( 'NONE',  ( -0.0004442498508594591917, 0.001194404164628348752, -65.00000000000000000 ) ) ;
#29353=CARTESIAN_POINT ( 'NONE',  ( -0.0004442498508594591917, 0.001194404164628348752, -65.00000000000000000 ) ) ;
#29541=VERTEX_POINT ( 'NONE', #11158 ) ;
#29601=VERTEX_POINT ( 'NONE', #74305 ) ;
#29830=ORIENTED_EDGE ( 'NONE', *, *, #62402, .F. ) ;
#29848=FACE_OUTER_BOUND ( 'NONE', #15906, .T. ) ;
#29994=DIRECTION ( 'NONE',  ( 7.705842312279274921E-15, -1.000000000000000000, 2.546204323184492723E-14 ) ) ;
#30006=CYLINDRICAL_SURFACE ( 'NONE', #55268, 12.75000000000265565 ) ;
#30017=CIRCLE ( 'NONE', #72047, 2.650000000000540812 ) ;
#30064=PLANE ( 'NONE',  #72149 ) ;
#30104=CYLINDRICAL_SURFACE ( 'NONE', #35338, 26.50000000000552092 ) ;
#30147=SHAPE_DEFINITION_REPRESENTATION ( #9143, #67135 ) ;
#30181=CARTESIAN_POINT ( 'NONE',  ( 2.184357737007946383E-12, -120.0000000000000000, -48.99999999999997158 ) ) ;
#30205=EDGE_CURVE ( 'NONE', #18161, #63726, #33433, .T. ) ;
#30337=ORIENTED_EDGE ( 'NONE', *, *, #50859, .F. ) ;
#30357=CARTESIAN_POINT ( 'NONE',  ( -0.0004442498507136653329, 0.001194404164628348752, -70.59999999999999432 ) ) ;
#30366=DIRECTION ( 'NONE',  ( 1.000000000000000000, -1.047380211910311281E-14, -2.618450529775778123E-14 ) ) ;
#30391=PRESENTATION_STYLE_ASSIGNMENT (( #24039 ) ) ;
#30402=DIRECTION ( 'NONE',  ( -2.603472992745699578E-14, 2.546204323184531851E-14, -1.000000000000000000 ) ) ;
#30434=FACE_OUTER_BOUND ( 'NONE', #14441, .T. ) ;
#30448=DIRECTION ( 'NONE',  ( -2.603472992746261562E-14, -2.546204323184492723E-14, 1.000000000000000000 ) ) ;
#30495=EDGE_LOOP ( 'NONE', ( #22561, #33556 ) ) ;
#30622=ORIENTED_EDGE ( 'NONE', *, *, #51935, .F. ) ;
#30632=EDGE_CURVE ( 'NONE', #17145, #63489, #41875, .T. ) ;
#30639=DIRECTION ( 'NONE',  ( 2.603472992746261562E-14, 2.546204323184492723E-14, -1.000000000000000000 ) ) ;
#30682=VERTEX_POINT ( 'NONE', #10887 ) ;
#30711=VERTEX_POINT ( 'NONE', #19101 ) ;
#30765=ORIENTED_EDGE ( 'NONE', *, *, #51367, .T. ) ;
#30873=ORIENTED_EDGE ( 'NONE', *, *, #5612, .F. ) ;
#31029=VECTOR ( 'NONE', #3141, 1000.000000000000000 ) ;
#31179=CARTESIAN_POINT ( 'NONE',  ( -95.00000000002611955, 90.00000000000007105, -75.00000000000000000 ) ) ;
#31185=CARTESIAN_POINT ( 'NONE',  ( -97.65000000002615366, -210.0000000000000284, -64.99999999999356248 ) ) ;
#31261=EDGE_LOOP ( 'NONE', ( #24145, #38755 ) ) ;
#31330=CARTESIAN_POINT ( 'NONE',  ( -95.00000000002611955, 90.00000000000007105, -75.00000000000000000 ) ) ;
#31376=DIRECTION ( 'NONE',  ( 1.000000000000000000, -7.677074106448950501E-15, -2.598394312951952234E-14 ) ) ;
#31378=EDGE_CURVE ( 'NONE', #35409, #30682, #38813, .T. ) ;
#31419=CARTESIAN_POINT ( 'NONE',  ( -97.65000000002672209, -209.9999999999999147, -74.99999999999342037 ) ) ;
#31443=EDGE_LOOP ( 'NONE', ( #59961, #42989, #15970, #353 ) ) ;
#31501=CIRCLE ( 'NONE', #8715, 15.70000000000326956 ) ;
#31522=VERTEX_POINT ( 'NONE', #57957 ) ;
#31523=CARTESIAN_POINT ( 'NONE',  ( -0.0004442498512760095037, 0.001194404164628348752, -49.00000000000000000 ) ) ;
#31551=PRODUCT_DEFINITION ( 'UNKNOWN', '', #58026, #31850 ) ;
#31591=CIRCLE ( 'NONE', #42405, 2.650000000000540812 ) ;
#31664=DIRECTION ( 'NONE',  ( 2.603472992746261562E-14, 2.546204323184492723E-14, -1.000000000000000000 ) ) ;
#31703=ORIENTED_EDGE ( 'NONE', *, *, #6562, .F. ) ;
#31738=ORIENTED_EDGE ( 'NONE', *, *, #25485, .T. ) ;
#31757=DIRECTION ( 'NONE',  ( -1.000000000000000000, -7.616308197389468785E-15, 2.603472992745757322E-14 ) ) ;
#31846=CARTESIAN_POINT ( 'NONE',  ( 100.0000000000260201, 95.00000000000001421, 74.99999999999998579 ) ) ;
#31850=PRODUCT_DEFINITION_CONTEXT ( 'detailed design', #53241, 'design' ) ;
#31870=CYLINDRICAL_SURFACE ( 'NONE', #48870, 15.70000000000326956 ) ;
#31906=DIRECTION ( 'NONE',  ( 1.000000000000000000, -3.961972362386988449E-13, -2.612289469705706555E-14 ) ) ;
#31938=CIRCLE ( 'NONE', #47570, 26.50000000000552092 ) ;
#31951=EDGE_LOOP ( 'NONE', ( #39650, #15630, #66416, #68252 ) ) ;
#31997=CARTESIAN_POINT ( 'NONE',  ( 12.74955575014913833, 0.001194404169505926478, -64.99999999999967315 ) ) ;
#32137=CYLINDRICAL_SURFACE ( 'NONE', #17865, 15.70000000000326956 ) ;
#32262=VERTEX_POINT ( 'NONE', #56592 ) ;
#32266=AXIS2_PLACEMENT_3D ( 'NONE', #55792, #10297, #62945 ) ;
#32268=CARTESIAN_POINT ( 'NONE',  ( 2.600855584879231068E-12, -120.0000000000000000, -65.00000000000000000 ) ) ;
#32298=CARTESIAN_POINT ( 'NONE',  ( 95.00000000002596323, -209.9999999999999147, -74.99999999999349143 ) ) ;
#32301=DIRECTION ( 'NONE',  ( -7.705842312279274921E-15, 1.000000000000000000, -2.546204323184492723E-14 ) ) ;
#32409=LINE ( 'NONE', #2785, #31029 ) ;
#32420=EDGE_CURVE ( 'NONE', #30682, #15051, #11782, .T. ) ;
#32476=EDGE_LOOP ( 'NONE', ( #36483, #72569, #31738, #62814 ) ) ;
#32544=DIRECTION ( 'NONE',  ( 2.603472992746261562E-14, 2.546204323184492723E-14, -1.000000000000000000 ) ) ;
#32569=CARTESIAN_POINT ( 'NONE',  ( 23.49955575014914189, 0.001194404164656991856, -64.99999999999938893 ) ) ;
#32850=FACE_BOUND ( 'NONE', #69127, .T. ) ;
#32889=DIRECTION ( 'NONE',  ( -1.000000000000000000, 7.619177619974977057E-15, 2.612289469705706555E-14 ) ) ;
#32907=DIRECTION ( 'NONE',  ( -2.603472992746261562E-14, -2.546204323184492723E-14, 1.000000000000000000 ) ) ;
#32910=ORIENTED_EDGE ( 'NONE', *, *, #69605, .F. ) ;
#32956=CYLINDRICAL_SURFACE ( 'NONE', #42014, 23.50000000000489919 ) ;
#32959=CARTESIAN_POINT ( 'NONE',  ( -15.70044424985398557, 0.001194404164747221980, -70.59999999999959641 ) ) ;
#33064=ADVANCED_FACE ( 'NONE', ( #50747, #3801 ), #67682, .T. ) ;
#33117=CARTESIAN_POINT ( 'NONE',  ( 15.70000000000602114, -120.0000000000001137, -70.60000000000039222 ) ) ;
#33149=DIRECTION ( 'NONE',  ( -1.000000000000000000, 7.955419762439749020E-15, 2.563413034563919251E-14 ) ) ;
#33184=CARTESIAN_POINT ( 'NONE',  ( -26.49999999999781863, -119.9999999999996021, -49.00000000000066080 ) ) ;
#33218=LINE ( 'NONE', #5427, #71503 ) ;
#33240=CARTESIAN_POINT ( 'NONE',  ( -0.0004442498508594591917, 0.001194404164628348752, -65.00000000000000000 ) ) ;
#33250=DIRECTION ( 'NONE',  ( -1.000000000000000000, 7.571543891232750625E-15, 2.563413034563919882E-14 ) ) ;
#33382=FACE_OUTER_BOUND ( 'NONE', #37169, .T. ) ;
#33393=ORIENTED_EDGE ( 'NONE', *, *, #69910, .T. ) ;
#33433=CIRCLE ( 'NONE', #46655, 26.50000000000552092 ) ;
#33556=ORIENTED_EDGE ( 'NONE', *, *, #50505, .F. ) ;
#33566=CARTESIAN_POINT ( 'NONE',  ( -23.49999999999740297, -119.9999999999996021, -65.00000000000061107 ) ) ;
#33789=FACE_BOUND ( 'NONE', #39218, .T. ) ;
#33876=MECHANICAL_DESIGN_GEOMETRIC_PRESENTATION_REPRESENTATION('',(#47083),#68715);
#33923=VECTOR ( 'NONE', #73851, 1000.000000000000000 ) ;
#33939=ORIENTED_EDGE ( 'NONE', *, *, #67968, .F. ) ;
#33967=FACE_OUTER_BOUND ( 'NONE', #67517, .T. ) ;
#33989=LINE ( 'NONE', #50537, #74243 ) ;
#34100=AXIS2_PLACEMENT_3D ( 'NONE', #49050, #30639, #26495 ) ;
#34264=AXIS2_PLACEMENT_3D ( 'NONE', #68669, #11501, #1388 ) ;
#34280=ORIENTED_EDGE ( 'NONE', *, *, #29009, .T. ) ;
#34343=FACE_BOUND ( 'NONE', #30495, .T. ) ;
#34504=CYLINDRICAL_SURFACE ( 'NONE', #55239, 12.75000000000265388 ) ;
#34517=ORIENTED_EDGE ( 'NONE', *, *, #70284, .F. ) ;
#34521=CARTESIAN_POINT ( 'NONE',  ( -26.50044424985086522, 0.001194404165032690894, -65.00000000000069633 ) ) ;
#34533=FACE_OUTER_BOUND ( 'NONE', #66851, .T. ) ;
#34581=ORIENTED_EDGE ( 'NONE', *, *, #28113, .T. ) ;
#34598=AXIS2_PLACEMENT_3D ( 'NONE', #17462, #52038, #23477 ) ;
#34612=DIRECTION ( 'NONE',  ( 1.000000000000000000, -7.571537405616606460E-15, -2.598394312951952234E-14 ) ) ;
#34719=DIRECTION ( 'NONE',  ( 1.000000000000000000, -1.047380211910311281E-14, -2.618450529775778123E-14 ) ) ;
#34816=AXIS2_PLACEMENT_3D ( 'NONE', #18334, #36734, #36362 ) ;
#34894=ORIENTED_EDGE ( 'NONE', *, *, #7414, .T. ) ;
#34919=DIRECTION ( 'NONE',  ( -1.000000000000000000, 7.331661483372147883E-15, 2.592266024478009537E-14 ) ) ;
#34940=DIRECTION ( 'NONE',  ( -2.603472992746261562E-14, -2.546204323184492723E-14, 1.000000000000000000 ) ) ;
#35090=CARTESIAN_POINT ( 'NONE',  ( -95.00000000002611955, 90.00000000000007105, -75.00000000000000000 ) ) ;
#35155=CARTESIAN_POINT ( 'NONE',  ( 97.65000000002596892, -210.0000000000000853, -64.99999999999342037 ) ) ;
#35212=ADVANCED_FACE ( 'NONE', ( #62782 ), #23639, .F. ) ;
#35288=CARTESIAN_POINT ( 'NONE',  ( -0.0004442498558709490585, 0.001194404164628348752, 127.4927882439603195 ) ) ;
#35304=CARTESIAN_POINT ( 'NONE',  ( 2.746650072473138780E-12, -120.0000000000000000, -70.59999999999999432 ) ) ;
#35331=EDGE_LOOP ( 'NONE', ( #30873, #25793 ) ) ;
#35338=AXIS2_PLACEMENT_3D ( 'NONE', #58691, #5726, #35392 ) ;
#35392=DIRECTION ( 'NONE',  ( -1.000000000000000000, 7.331661483372147883E-15, 2.592266024478009537E-14 ) ) ;
#35409=VERTEX_POINT ( 'NONE', #32959 ) ;
#35420=ORIENTED_EDGE ( 'NONE', *, *, #49306, .T. ) ;
#35522=EDGE_LOOP ( 'NONE', ( #21365, #25791 ) ) ;
#35565=CARTESIAN_POINT ( 'NONE',  ( -15.70000000000052687, -119.9999999999998721, -70.59999999999959641 ) ) ;
#35591=SHAPE_REPRESENTATION_RELATIONSHIP ( 'NONE' , 'NONE' ,  #67135, #13932 ) ;
#35660=VERTEX_POINT ( 'NONE', #36671 ) ;
#35744=AXIS2_PLACEMENT_3D ( 'NONE', #44068, #31664, #54609 ) ;
#35767=CIRCLE ( 'NONE', #20153, 2.650000000000540812 ) ;
#35901=VECTOR ( 'NONE', #42557, 1000.000000000000000 ) ;
#35927=CIRCLE ( 'NONE', #73106, 12.75000000000265388 ) ;
#35953=AXIS2_PLACEMENT_3D ( 'NONE', #31179, #53384, #47736 ) ;
#35997=CARTESIAN_POINT ( 'NONE',  ( -0.0004442498512760095037, 0.001194404164628348752, -49.00000000000000000 ) ) ;
#36040=CARTESIAN_POINT ( 'NONE',  ( 2.184357737007946383E-12, -120.0000000000000000, -48.99999999999997158 ) ) ;
#36362=DIRECTION ( 'NONE',  ( -1.000000000000000000, 1.047380211910311281E-14, 2.618450529775778123E-14 ) ) ;
#36479=ADVANCED_FACE ( 'NONE', ( #56847 ), #56483, .F. ) ;
#36483=ORIENTED_EDGE ( 'NONE', *, *, #51725, .F. ) ;
#36575=EDGE_CURVE ( 'NONE', #58103, #18206, #44167, .T. ) ;
#36617=AXIS2_PLACEMENT_3D ( 'NONE', #18554, #13284, #53514 ) ;
#36671=CARTESIAN_POINT ( 'NONE',  ( -12.75044424985085634, 0.001194404169697439516, -65.00000000000034106 ) ) ;
#36734=DIRECTION ( 'NONE',  ( 2.603472992746261562E-14, 2.546204323184492723E-14, -1.000000000000000000 ) ) ;
#36743=EDGE_CURVE ( 'NONE', #46060, #37710, #36860, .T. ) ;
#36780=DIRECTION ( 'NONE',  ( 1.000000000000000000, -5.236901059551556403E-15, -2.618450529775778123E-14 ) ) ;
#36844=UNCERTAINTY_MEASURE_WITH_UNIT (LENGTH_MEASURE( 1.000000000000000082E-05 ), #18373, 'distance_accuracy_value', 'NONE');
#36860=LINE ( 'NONE', #15035, #46633 ) ;
#36863=CARTESIAN_POINT ( 'NONE',  ( -92.35000000002557385, 90.00000000000005684, -75.00000000000007105 ) ) ;
#36924=DIRECTION ( 'NONE',  ( -2.603472992746261562E-14, -2.546204323184492723E-14, 1.000000000000000000 ) ) ;
#36937=LINE ( 'NONE', #41473, #12814 ) ;
#36965=ORIENTED_EDGE ( 'NONE', *, *, #23932, .T. ) ;
#36969=ORIENTED_EDGE ( 'NONE', *, *, #67476, .F. ) ;
#37099=ADVANCED_FACE ( 'NONE', ( #54716 ), #32137, .F. ) ;
#37131=AXIS2_PLACEMENT_3D ( 'NONE', #31523, #28476, #339 ) ;
#37141=DIRECTION ( 'NONE',  ( 2.603472992746261562E-14, 2.546204323184492723E-14, -1.000000000000000000 ) ) ;
#37169=EDGE_LOOP ( 'NONE', ( #19942, #64267, #50603, #22177 ) ) ;
#37187=FACE_OUTER_BOUND ( 'NONE', #31951, .T. ) ;
#37392=EDGE_LOOP ( 'NONE', ( #55074, #24758, #19688, #27273 ) ) ;
#37485=( GEOMETRIC_REPRESENTATION_CONTEXT ( 3 ) GLOBAL_UNCERTAINTY_ASSIGNED_CONTEXT ( ( #20295 ) ) GLOBAL_UNIT_ASSIGNED_CONTEXT ( ( #44678, #5204, #39776 ) ) REPRESENTATION_CONTEXT ( 'NONE', 'WORKASPACE' ) );
#37597=DIRECTION ( 'NONE',  ( 7.705842312279274921E-15, -1.000000000000000000, 2.546204323184492723E-14 ) ) ;
#37710=VERTEX_POINT ( 'NONE', #27526 ) ;
#37721=ORIENTED_EDGE ( 'NONE', *, *, #6798, .T. ) ;
#37814=EDGE_LOOP ( 'NONE', ( #62826, #73441 ) ) ;
#37877=DIRECTION ( 'NONE',  ( 2.603472992746261562E-14, 2.546204323184492723E-14, -1.000000000000000000 ) ) ;
#37945=ORIENTED_EDGE ( 'NONE', *, *, #23292, .F. ) ;
#37977=DIRECTION ( 'NONE',  ( 2.603472992746261562E-14, 2.546204323184492723E-14, -1.000000000000000000 ) ) ;
#38019=LINE ( 'NONE', #20361, #35901 ) ;
#38091=ORIENTED_EDGE ( 'NONE', *, *, #49422, .F. ) ;
#38137=MANIFOLD_SOLID_BREP ( 'M5 Clearance Hole1', #40409 ) ;
#38224=ORIENTED_EDGE ( 'NONE', *, *, #40834, .F. ) ;
#38258=EDGE_CURVE ( 'NONE', #25904, #54110, #63228, .T. ) ;
#38365=DIRECTION ( 'NONE',  ( 1.000000000000000000, -7.571541139944063212E-15, -2.603472992745718826E-14 ) ) ;
#38388=ADVANCED_FACE ( 'NONE', ( #65731 ), #31870, .F. ) ;
#38414=EDGE_LOOP ( 'NONE', ( #52671, #47345, #15468, #34517 ) ) ;
#38508=DIRECTION ( 'NONE',  ( 1.000000000000000000, -7.571541139944063212E-15, -2.603472992745718826E-14 ) ) ;
#38514=ADVANCED_FACE ( 'NONE', ( #74330 ), #61946, .T. ) ;
#38755=ORIENTED_EDGE ( 'NONE', *, *, #70585, .F. ) ;
#38813=LINE ( 'NONE', #39186, #25191 ) ;
#38880=FACE_BOUND ( 'NONE', #31261, .T. ) ;
#39172=DIRECTION ( 'NONE',  ( 2.603472992746261562E-14, 2.546204323184492723E-14, -1.000000000000000000 ) ) ;
#39186=CARTESIAN_POINT ( 'NONE',  ( -15.70044424985398557, 0.001194404164747221980, -70.59999999999959641 ) ) ;
#39218=EDGE_LOOP ( 'NONE', ( #70261, #14786 ) ) ;
#39227=DIRECTION ( 'NONE',  ( -2.603472992746261562E-14, -2.546204323184492723E-14, 1.000000000000000000 ) ) ;
#39398=CARTESIAN_POINT ( 'NONE',  ( 26.49955575015424358, 0.001194404164430948063, -49.00000000000068923 ) ) ;
#39441=LINE ( 'NONE', #21375, #665 ) ;
#39518=LINE ( 'NONE', #63565, #70688 ) ;
#39527=CIRCLE ( 'NONE', #17885, 2.650000000000540812 ) ;
#39555=DIRECTION ( 'NONE',  ( 2.603472992746261562E-14, 2.546204323184492723E-14, -1.000000000000000000 ) ) ;
#39583=EDGE_LOOP ( 'NONE', ( #60868, #34894, #28110, #30622 ) ) ;
#39650=ORIENTED_EDGE ( 'NONE', *, *, #48541, .T. ) ;
#39776=( NAMED_UNIT ( * ) SI_UNIT ( $, .STERADIAN. ) SOLID_ANGLE_UNIT ( ) );
#39835=CARTESIAN_POINT ( 'NONE',  ( -95.00000000002617639, -209.9999999999999432, -74.99999999999349143 ) ) ;
#40090=ADVANCED_FACE ( 'NONE', ( #22573, #6399 ), #17666, .T. ) ;
#40137=SURFACE_SIDE_STYLE ('',( #17206 ) ) ;
#40207=AXIS2_PLACEMENT_3D ( 'NONE', #41612, #12296, #41996 ) ;
#40261=CARTESIAN_POINT ( 'NONE',  ( 95.00000000002596323, -209.9999999999999147, -74.99999999999349143 ) ) ;
#40286=VERTEX_POINT ( 'NONE', #13501 ) ;
#40291=FACE_OUTER_BOUND ( 'NONE', #64459, .T. ) ;
#40303=CARTESIAN_POINT ( 'NONE',  ( -23.50044424985617653, 0.001194404164806279773, -48.99999999999938893 ) ) ;
#40409=CLOSED_SHELL ( 'NONE', ( #55999, #57791, #52458, #10892, #67933, #37099, #40564, #53920, #56864, #29122, #35212, #15882, #2442, #72050, #33064, #4207, #7043, #47278, #68101, #36479, #21796, #27895, #8485, #52426, #1416, #41606, #38514, #2994, #38388, #40090, #24218, #62046, #11845, #48489, #11125, #63910 ) ) ;
#40445=CARTESIAN_POINT ( 'NONE',  ( -23.49999999999781863, -119.9999999999996021, -49.00000000000058265 ) ) ;
#40564=ADVANCED_FACE ( 'NONE', ( #37187 ), #8610, .F. ) ;
#40651=DIRECTION ( 'NONE',  ( -2.603472992746261562E-14, -2.546204323184492723E-14, 1.000000000000000000 ) ) ;
#40682=ORIENTED_EDGE ( 'NONE', *, *, #71955, .F. ) ;
#40738=FACE_BOUND ( 'NONE', #24259, .T. ) ;
#40834=EDGE_CURVE ( 'NONE', #25604, #6768, #48382, .T. ) ;
#41200=EDGE_CURVE ( 'NONE', #14031, #44982, #13180, .T. ) ;
#41224=CIRCLE ( 'NONE', #5184, 2.650000000000540812 ) ;
#41305=DIRECTION ( 'NONE',  ( 2.603472992746261562E-14, 2.546204323184492723E-14, -1.000000000000000000 ) ) ;
#41354=ORIENTED_EDGE ( 'NONE', *, *, #48450, .T. ) ;
#41473=CARTESIAN_POINT ( 'NONE',  ( -12.75044424985852487, 0.001194404164724885897, 127.4927882439606464 ) ) ;
#41500=ORIENTED_EDGE ( 'NONE', *, *, #27260, .T. ) ;
#41551=DIRECTION ( 'NONE',  ( 2.603472992745699578E-14, -2.546204323184531851E-14, 1.000000000000000000 ) ) ;
#41606=ADVANCED_FACE ( 'NONE', ( #33967, #57277 ), #27586, .T. ) ;
#41612=CARTESIAN_POINT ( 'NONE',  ( 2.746650072473138780E-12, -120.0000000000000000, -70.59999999999999432 ) ) ;
#41691=CARTESIAN_POINT ( 'NONE',  ( 2.746707903440850533E-12, -120.0000000000000000, -70.59999999999999432 ) ) ;
#41758=DIRECTION ( 'NONE',  ( -1.000000000000000000, 7.571543891232750625E-15, 2.563413034563919882E-14 ) ) ;
#41813=CARTESIAN_POINT ( 'NONE',  ( -92.35000000002618492, -210.0000000000000853, -74.99999999999342037 ) ) ;
#41853=EDGE_CURVE ( 'NONE', #32262, #27633, #30017, .T. ) ;
#41875=CIRCLE ( 'NONE', #51476, 2.650000000000540812 ) ;
#41878=ORIENTED_EDGE ( 'NONE', *, *, #10250, .F. ) ;
#41930=CARTESIAN_POINT ( 'NONE',  ( 23.49955575014872622, 0.001194404164656991856, -48.99999999999938893 ) ) ;
#41996=DIRECTION ( 'NONE',  ( -1.000000000000000000, 7.619177619974977057E-15, 2.612289469705706555E-14 ) ) ;
#42014=AXIS2_PLACEMENT_3D ( 'NONE', #62299, #15684, #12534 ) ;
#42054=EDGE_CURVE ( 'NONE', #35660, #46991, #35927, .T. ) ;
#42105=DIRECTION ( 'NONE',  ( 2.603472992746261562E-14, 2.546204323184492723E-14, -1.000000000000000000 ) ) ;
#42388=FACE_OUTER_BOUND ( 'NONE', #5570, .T. ) ;
#42405=AXIS2_PLACEMENT_3D ( 'NONE', #51364, #58123, #45757 ) ;
#42522=VERTEX_POINT ( 'NONE', #27212 ) ;
#42557=DIRECTION ( 'NONE',  ( 2.603472992746261562E-14, 2.546204323184492723E-14, -1.000000000000000000 ) ) ;
#42575=ORIENTED_EDGE ( 'NONE', *, *, #23932, .F. ) ;
#42578=CARTESIAN_POINT ( 'NONE',  ( 95.00000000002597744, 90.00000000000007105, -65.00000000000000000 ) ) ;
#42815=ORIENTED_EDGE ( 'NONE', *, *, #19451, .F. ) ;
#42890=EDGE_CURVE ( 'NONE', #63489, #17145, #35767, .T. ) ;
#42945=EDGE_CURVE ( 'NONE', #17492, #59102, #24942, .T. ) ;
#42989=ORIENTED_EDGE ( 'NONE', *, *, #36575, .F. ) ;
#43013=VERTEX_POINT ( 'NONE', #52763 ) ;
#43094=AXIS2_PLACEMENT_3D ( 'NONE', #52672, #7920, #41758 ) ;
#43223=ORIENTED_EDGE ( 'NONE', *, *, #38258, .F. ) ;
#43360=AXIS2_PLACEMENT_3D ( 'NONE', #15378, #71771, #43610 ) ;
#43395=AXIS2_PLACEMENT_3D ( 'NONE', #48320, #71232, #19735 ) ;
#43610=DIRECTION ( 'NONE',  ( -1.000000000000000000, 1.047380211910311281E-14, 2.618450529775778123E-14 ) ) ;
#43668=ORIENTED_EDGE ( 'NONE', *, *, #30632, .F. ) ;
#43719=CARTESIAN_POINT ( 'NONE',  ( -0.0004442498505991059293, 0.001194404164628348752, -75.00000000000000000 ) ) ;
#43795=DIRECTION ( 'NONE',  ( -2.603472992746261562E-14, -2.546204323184492723E-14, 1.000000000000000000 ) ) ;
#43802=FACE_OUTER_BOUND ( 'NONE', #72345, .T. ) ;
#43811=CARTESIAN_POINT ( 'NONE',  ( 100.0000000000260201, 95.00000000000001421, 74.99999999999998579 ) ) ;
#44068=CARTESIAN_POINT ( 'NONE',  ( -0.0004442498507136653329, 0.001194404164628348752, -70.59999999999999432 ) ) ;
#44071=EDGE_CURVE ( 'NONE', #63658, #35409, #8245, .T. ) ;
#44167=CIRCLE ( 'NONE', #24945, 15.70000000000327312 ) ;
#44237=EDGE_CURVE ( 'NONE', #49091, #53076, #20306, .T. ) ;
#44536=DIRECTION ( 'NONE',  ( -2.603472992746261562E-14, -2.546204323184492723E-14, 1.000000000000000000 ) ) ;
#44678=( LENGTH_UNIT ( ) NAMED_UNIT ( * ) SI_UNIT ( .MILLI., .METRE. ) );
#44738=AXIS2_PLACEMENT_3D ( 'NONE', #28324, #27593, #38508 ) ;
#44757=ORIENTED_EDGE ( 'NONE', *, *, #49306, .F. ) ;
#44842=ORIENTED_EDGE ( 'NONE', *, *, #36575, .T. ) ;
#44884=CARTESIAN_POINT ( 'NONE',  ( 2.600913415846943225E-12, -120.0000000000000000, -65.00000000000000000 ) ) ;
#44982=VERTEX_POINT ( 'NONE', #61938 ) ;
#45309=ORIENTED_EDGE ( 'NONE', *, *, #30632, .T. ) ;
#45407=DIRECTION ( 'NONE',  ( 2.603472992746261562E-14, 2.546204323184492723E-14, -1.000000000000000000 ) ) ;
#45524=EDGE_CURVE ( 'NONE', #10395, #75, #48157, .T. ) ;
#45594=DIRECTION ( 'NONE',  ( 2.603472992746261562E-14, 2.546204323184492723E-14, -1.000000000000000000 ) ) ;
#45621=CIRCLE ( 'NONE', #63598, 23.50000000000489919 ) ;
#45653=FACE_OUTER_BOUND ( 'NONE', #61848, .T. ) ;
#45664=AXIS2_PLACEMENT_3D ( 'NONE', #32268, #8981, #31906 ) ;
#45688=LINE ( 'NONE', #57697, #33923 ) ;
#45757=DIRECTION ( 'NONE',  ( -1.000000000000000000, 5.236901059551556403E-15, 2.618450529775778123E-14 ) ) ;
#45771=ORIENTED_EDGE ( 'NONE', *, *, #12634, .F. ) ;
#45923=EDGE_CURVE ( 'NONE', #27633, #32262, #19079, .T. ) ;
#46008=EDGE_CURVE ( 'NONE', #62552, #53187, #45621, .T. ) ;
#46060=VERTEX_POINT ( 'NONE', #22015 ) ;
#46112=EDGE_CURVE ( 'NONE', #2456, #7432, #9626, .T. ) ;
#46205=FACE_OUTER_BOUND ( 'NONE', #12779, .T. ) ;
#46218=DIRECTION ( 'NONE',  ( 2.603472992746261562E-14, 2.546204323184492723E-14, -1.000000000000000000 ) ) ;
#46237=DIRECTION ( 'NONE',  ( -1.000000000000000000, 7.571541139944063212E-15, 2.603472992745718826E-14 ) ) ;
#46299=CIRCLE ( 'NONE', #34264, 15.70000000000327312 ) ;
#46348=CIRCLE ( 'NONE', #767, 26.50000000000552092 ) ;
#46357=DIRECTION ( 'NONE',  ( 2.603472992746261562E-14, 2.546204323184492723E-14, -1.000000000000000000 ) ) ;
#46441=EDGE_LOOP ( 'NONE', ( #33939, #21710 ) ) ;
#46481=DIRECTION ( 'NONE',  ( 1.000000000000000000, -7.619177619974977057E-15, -2.612289469705706555E-14 ) ) ;
#46513=( LENGTH_UNIT ( ) NAMED_UNIT ( * ) SI_UNIT ( .MILLI., .METRE. ) );
#46569=DIRECTION ( 'NONE',  ( 2.603472992746261562E-14, 2.546204323184492723E-14, -1.000000000000000000 ) ) ;
#46633=VECTOR ( 'NONE', #37977, 1000.000000000000000 ) ;
#46655=AXIS2_PLACEMENT_3D ( 'NONE', #840, #40651, #23723 ) ;
#46691=ORIENTED_EDGE ( 'NONE', *, *, #70318, .F. ) ;
#46716=AXIS2_PLACEMENT_3D ( 'NONE', #32298, #66896, #4891 ) ;
#46775=CYLINDRICAL_SURFACE ( 'NONE', #36617, 2.650000000000540812 ) ;
#46868=EDGE_LOOP ( 'NONE', ( #55336, #13870 ) ) ;
#46916=CARTESIAN_POINT ( 'NONE',  ( 100.0000000000260201, 95.00000000000001421, -65.00000000000001421 ) ) ;
#46988=ORIENTED_EDGE ( 'NONE', *, *, #6484, .F. ) ;
#46991=VERTEX_POINT ( 'NONE', #31997 ) ;
#47051=AXIS2_PLACEMENT_3D ( 'NONE', #11179, #55560, #49905 ) ;
#47082=EDGE_LOOP ( 'NONE', ( #42815, #73811, #52083, #70189 ) ) ;
#47083=STYLED_ITEM ( 'NONE', ( #28852 ), #13932 ) ;
#47165=CYLINDRICAL_SURFACE ( 'NONE', #56075, 26.50000000000552092 ) ;
#47199=FACE_BOUND ( 'NONE', #46441, .T. ) ;
#47278=ADVANCED_FACE ( 'NONE', ( #47729 ), #30064, .F. ) ;
#47345=ORIENTED_EDGE ( 'NONE', *, *, #6562, .T. ) ;
#47403=DIRECTION ( 'NONE',  ( -2.603472992746261562E-14, -2.546204323184492723E-14, 1.000000000000000000 ) ) ;
#47479=DIRECTION ( 'NONE',  ( 2.603472992746261562E-14, 2.546204323184492723E-14, -1.000000000000000000 ) ) ;
#47519=ORIENTED_EDGE ( 'NONE', *, *, #58712, .F. ) ;
#47540=DIRECTION ( 'NONE',  ( -2.603472992746261562E-14, -2.546204323184492723E-14, 1.000000000000000000 ) ) ;
#47570=AXIS2_PLACEMENT_3D ( 'NONE', #44884, #74179, #61055 ) ;
#47703=PLANE ( 'NONE',  #66980 ) ;
#47727=ORIENTED_EDGE ( 'NONE', *, *, #51700, .F. ) ;
#47729=FACE_OUTER_BOUND ( 'NONE', #38414, .T. ) ;
#47736=DIRECTION ( 'NONE',  ( -1.000000000000000000, 5.236901059551556403E-15, 2.618450529775778123E-14 ) ) ;
#47754=AXIS2_PLACEMENT_3D ( 'NONE', #50065, #10227, #17356 ) ;
#47760=CARTESIAN_POINT ( 'NONE',  ( 97.65000000002650893, -209.9999999999999432, -74.99999999999356248 ) ) ;
#47930=ORIENTED_EDGE ( 'NONE', *, *, #5362, .F. ) ;
#47936=DIRECTION ( 'NONE',  ( -2.603472992746261562E-14, -2.546204323184492723E-14, 1.000000000000000000 ) ) ;
#47994=ORIENTED_EDGE ( 'NONE', *, *, #30205, .T. ) ;
#47995=AXIS2_PLACEMENT_3D ( 'NONE', #15198, #47936, #31376 ) ;
#48097=VERTEX_POINT ( 'NONE', #14362 ) ;
#48135=FACE_OUTER_BOUND ( 'NONE', #37392, .T. ) ;
#48157=LINE ( 'NONE', #36863, #7116 ) ;
#48320=CARTESIAN_POINT ( 'NONE',  ( 0.000000000000000000, 0.000000000000000000, 0.000000000000000000 ) ) ;
#48363=CARTESIAN_POINT ( 'NONE',  ( 100.0000000000260343, -214.9999999999999716, -64.99999999999350564 ) ) ;
#48382=LINE ( 'NONE', #46916, #57583 ) ;
#48405=DIRECTION ( 'NONE',  ( -2.603472992746261562E-14, -2.546204323184492723E-14, 1.000000000000000000 ) ) ;
#48450=EDGE_CURVE ( 'NONE', #48097, #53076, #61486, .T. ) ;
#48489=ADVANCED_FACE ( 'NONE', ( #17330 ), #452, .F. ) ;
#48541=EDGE_CURVE ( 'NONE', #67107, #49091, #50633, .T. ) ;
#48567=ORIENTED_EDGE ( 'NONE', *, *, #13580, .T. ) ;
#48728=CARTESIAN_POINT ( 'NONE',  ( -97.65000000002672209, -209.9999999999999147, -74.99999999999342037 ) ) ;
#48858=CARTESIAN_POINT ( 'NONE',  ( -100.0000000000260485, 95.00000000000001421, -75.00000000000000000 ) ) ;
#48870=AXIS2_PLACEMENT_3D ( 'NONE', #55185, #54814, #3340 ) ;
#48871=LINE ( 'NONE', #47760, #56861 ) ;
#49047=DIRECTION ( 'NONE',  ( -2.603472992746261562E-14, -2.546204323184492723E-14, 1.000000000000000000 ) ) ;
#49050=CARTESIAN_POINT ( 'NONE',  ( 95.00000000002597744, 90.00000000000007105, -75.00000000000000000 ) ) ;
#49091=VERTEX_POINT ( 'NONE', #41930 ) ;
#49210=ORIENTED_EDGE ( 'NONE', *, *, #64926, .F. ) ;
#49306=EDGE_CURVE ( 'NONE', #59102, #17492, #25509, .T. ) ;
#49336=DIRECTION ( 'NONE',  ( 2.603472992746261562E-14, 2.546204323184492723E-14, -1.000000000000000000 ) ) ;
#49422=EDGE_CURVE ( 'NONE', #43013, #55201, #12317, .T. ) ;
#49471=CARTESIAN_POINT ( 'NONE',  ( 2.184357737007946383E-12, -120.0000000000000000, -48.99999999999997158 ) ) ;
#49741=CARTESIAN_POINT ( 'NONE',  ( 95.00000000002597744, 90.00000000000007105, -65.00000000000000000 ) ) ;
#49905=DIRECTION ( 'NONE',  ( 1.000000000000000000, -7.571537405616606460E-15, -2.598394312951952234E-14 ) ) ;
#49909=ORIENTED_EDGE ( 'NONE', *, *, #13580, .F. ) ;
#50011=VERTEX_POINT ( 'NONE', #70951 ) ;
#50065=CARTESIAN_POINT ( 'NONE',  ( -100.0000000000260059, -214.9999999999999716, 75.00000000001300293 ) ) ;
#50136=DIRECTION ( 'NONE',  ( -1.000000000000000000, 7.571543891232750625E-15, 2.563413034563919882E-14 ) ) ;
#50183=FACE_OUTER_BOUND ( 'NONE', #32476, .T. ) ;
#50226=EDGE_CURVE ( 'NONE', #62552, #17492, #4047, .T. ) ;
#50295=EDGE_LOOP ( 'NONE', ( #25033, #25518, #54082, #37721 ) ) ;
#50505=EDGE_CURVE ( 'NONE', #14126, #52133, #7703, .T. ) ;
#50537=CARTESIAN_POINT ( 'NONE',  ( 92.35000000002544596, 90.00000000000008527, -74.99999999999992895 ) ) ;
#50603=ORIENTED_EDGE ( 'NONE', *, *, #235, .T. ) ;
#50633=CIRCLE ( 'NONE', #47051, 23.50000000000489919 ) ;
#50649=CARTESIAN_POINT ( 'NONE',  ( -0.0004442498512760095037, 0.001194404164628348752, -49.00000000000000000 ) ) ;
#50747=FACE_BOUND ( 'NONE', #58147, .T. ) ;
#50758=DIRECTION ( 'NONE',  ( -1.000000000000000000, 7.571541139944063212E-15, 2.603472992745718826E-14 ) ) ;
#50780=CARTESIAN_POINT ( 'NONE',  ( 15.69955575014928328, 0.001194404164567414856, -70.59999999999959641 ) ) ;
#50859=EDGE_CURVE ( 'NONE', #20743, #73822, #7636, .T. ) ;
#50874=EDGE_LOOP ( 'NONE', ( #7314, #27368, #13036, #61598 ) ) ;
#51006=AXIS2_PLACEMENT_3D ( 'NONE', #35304, #46218, #69152 ) ;
#51036=ORIENTED_EDGE ( 'NONE', *, *, #42890, .T. ) ;
#51137=EDGE_LOOP ( 'NONE', ( #43668, #21616 ) ) ;
#51284=DIRECTION ( 'NONE',  ( 1.000000000000000000, -7.571537405616606460E-15, -2.598394312951952234E-14 ) ) ;
#51364=CARTESIAN_POINT ( 'NONE',  ( 95.00000000002597744, 90.00000000000007105, -75.00000000000000000 ) ) ;
#51367=EDGE_CURVE ( 'NONE', #55201, #56506, #48871, .T. ) ;
#51401=ORIENTED_EDGE ( 'NONE', *, *, #41853, .T. ) ;
#51476=AXIS2_PLACEMENT_3D ( 'NONE', #39835, #52572, #28527 ) ;
#51555=VECTOR ( 'NONE', #32544, 1000.000000000000000 ) ;
#51700=EDGE_CURVE ( 'NONE', #58103, #50011, #12627, .T. ) ;
#51702=CIRCLE ( 'NONE', #19280, 15.70000000000327312 ) ;
#51725=EDGE_CURVE ( 'NONE', #29601, #46060, #29196, .T. ) ;
#51759=LINE ( 'NONE', #309, #4779 ) ;
#51781=VERTEX_POINT ( 'NONE', #20860 ) ;
#51822=CARTESIAN_POINT ( 'NONE',  ( -100.0000000000260485, 95.00000000000001421, -75.00000000000000000 ) ) ;
#51935=EDGE_CURVE ( 'NONE', #53076, #48097, #73689, .T. ) ;
#51936=FACE_OUTER_BOUND ( 'NONE', #27469, .T. ) ;
#52038=DIRECTION ( 'NONE',  ( 2.603472992746261562E-14, 2.546204323184492723E-14, -1.000000000000000000 ) ) ;
#52083=ORIENTED_EDGE ( 'NONE', *, *, #69605, .T. ) ;
#52133=VERTEX_POINT ( 'NONE', #54979 ) ;
#52426=ADVANCED_FACE ( 'NONE', ( #51936 ), #30104, .T. ) ;
#52458=ADVANCED_FACE ( 'NONE', ( #40291 ), #24121, .F. ) ;
#52572=DIRECTION ( 'NONE',  ( 2.603472992746261562E-14, 2.546204323184492723E-14, -1.000000000000000000 ) ) ;
#52671=ORIENTED_EDGE ( 'NONE', *, *, #55071, .F. ) ;
#52672=CARTESIAN_POINT ( 'NONE',  ( -0.0004442498507136653329, 0.001194404164628348752, -70.59999999999999432 ) ) ;
#52763=CARTESIAN_POINT ( 'NONE',  ( 92.35000000002597176, -210.0000000000000284, -64.99999999999356248 ) ) ;
#52931=ORIENTED_EDGE ( 'NONE', *, *, #60584, .T. ) ;
#52973=EDGE_CURVE ( 'NONE', #37710, #31522, #69047, .T. ) ;
#53013=DIRECTION ( 'NONE',  ( 7.571541139946887334E-15, -1.000000000000000000, -2.546204323184473159E-14 ) ) ;
#53076=VERTEX_POINT ( 'NONE', #32569 ) ;
#53159=AXIS2_PLACEMENT_3D ( 'NONE', #17430, #30448, #34719 ) ;
#53187=VERTEX_POINT ( 'NONE', #40445 ) ;
#53211=AXIS2_PLACEMENT_3D ( 'NONE', #56218, #9970, #32889 ) ;
#53241=APPLICATION_CONTEXT ( 'automotive_design' ) ;
#53302=DIRECTION ( 'NONE',  ( 2.603472992746261562E-14, 2.546204323184492723E-14, -1.000000000000000000 ) ) ;
#53384=DIRECTION ( 'NONE',  ( 2.603472992746261562E-14, 2.546204323184492723E-14, -1.000000000000000000 ) ) ;
#53514=DIRECTION ( 'NONE',  ( -1.000000000000000000, 5.236901059551556403E-15, 2.618450529775778123E-14 ) ) ;
#53578=ORIENTED_EDGE ( 'NONE', *, *, #71520, .F. ) ;
#53651=DIRECTION ( 'NONE',  ( 2.603472992746261562E-14, 2.546204323184492723E-14, -1.000000000000000000 ) ) ;
#53661=EDGE_CURVE ( 'NONE', #67107, #48097, #17371, .T. ) ;
#53707=ORIENTED_EDGE ( 'NONE', *, *, #28113, .F. ) ;
#53920=ADVANCED_FACE ( 'NONE', ( #29848 ), #47165, .T. ) ;
#53926=CARTESIAN_POINT ( 'NONE',  ( -0.0004442498512760095037, 0.001194404164628348752, -49.00000000000000000 ) ) ;
#54072=DIRECTION ( 'NONE',  ( -1.000000000000000000, 7.619177619974977057E-15, 2.612289469705706555E-14 ) ) ;
#54082=ORIENTED_EDGE ( 'NONE', *, *, #9614, .T. ) ;
#54110=VERTEX_POINT ( 'NONE', #33184 ) ;
#54295=VECTOR ( 'NONE', #6234, 1000.000000000000000 ) ;
#54374=AXIS2_PLACEMENT_3D ( 'NONE', #53926, #47540, #2468 ) ;
#54586=VECTOR ( 'NONE', #37877, 1000.000000000000000 ) ;
#54609=DIRECTION ( 'NONE',  ( -1.000000000000000000, 7.571544473058805744E-15, 2.612289469705706870E-14 ) ) ;
#54614=AXIS2_PLACEMENT_3D ( 'NONE', #49741, #39227, #20811 ) ;
#54715=CIRCLE ( 'NONE', #22308, 2.650000000000540812 ) ;
#54716=FACE_OUTER_BOUND ( 'NONE', #58728, .T. ) ;
#54793=ORIENTED_EDGE ( 'NONE', *, *, #46008, .F. ) ;
#54814=DIRECTION ( 'NONE',  ( 2.603472992746261562E-14, 2.546204323184492723E-14, -1.000000000000000000 ) ) ;
#54856=ORIENTED_EDGE ( 'NONE', *, *, #63442, .F. ) ;
#54895=ORIENTED_EDGE ( 'NONE', *, *, #42945, .F. ) ;
#54973=VECTOR ( 'NONE', #39172, 1000.000000000000000 ) ;
#54979=CARTESIAN_POINT ( 'NONE',  ( 92.35000000002544596, 90.00000000000008527, -74.99999999999992895 ) ) ;
#55010=AXIS2_PLACEMENT_3D ( 'NONE', #55437, #49047, #71599 ) ;
#55071=EDGE_CURVE ( 'NONE', #6768, #42522, #7690, .T. ) ;
#55074=ORIENTED_EDGE ( 'NONE', *, *, #8906, .F. ) ;
#55185=CARTESIAN_POINT ( 'NONE',  ( -0.0004442498507136653329, 0.001194404164628348752, -70.59999999999999432 ) ) ;
#55201=VERTEX_POINT ( 'NONE', #35155 ) ;
#55239=AXIS2_PLACEMENT_3D ( 'NONE', #73241, #22500, #5224 ) ;
#55268=AXIS2_PLACEMENT_3D ( 'NONE', #25123, #41305, #54072 ) ;
#55336=ORIENTED_EDGE ( 'NONE', *, *, #45923, .F. ) ;
#55373=ORIENTED_EDGE ( 'NONE', *, *, #31378, .T. ) ;
#55434=DIRECTION ( 'NONE',  ( -1.000000000000000000, 7.955419762439749020E-15, 2.563413034563919251E-14 ) ) ;
#55437=CARTESIAN_POINT ( 'NONE',  ( -95.00000000002611955, 90.00000000000007105, -65.00000000000000000 ) ) ;
#55442=DIRECTION ( 'NONE',  ( 7.616308197390131428E-15, -1.000000000000000000, 2.546204323184492723E-14 ) ) ;
#55560=DIRECTION ( 'NONE',  ( -2.603472992746261562E-14, -2.546204323184492723E-14, 1.000000000000000000 ) ) ;
#55700=DIRECTION ( 'NONE',  ( 1.000000000000000000, -3.974818696583893186E-13, -2.612289469705706870E-14 ) ) ;
#55712=DIRECTION ( 'NONE',  ( 2.603472992746261562E-14, 2.546204323184492723E-14, -1.000000000000000000 ) ) ;
#55792=CARTESIAN_POINT ( 'NONE',  ( -0.0004442498512760095037, 0.001194404164628348752, -49.00000000000000000 ) ) ;
#55805=EDGE_LOOP ( 'NONE', ( #41354, #2842 ) ) ;
#55999=ADVANCED_FACE ( 'NONE', ( #34533 ), #69137, .F. ) ;
#56015=DIRECTION ( 'NONE',  ( 1.000000000000000000, -7.571544473058805744E-15, -2.612289469705706870E-14 ) ) ;
#56047=ORIENTED_EDGE ( 'NONE', *, *, #32420, .F. ) ;
#56065=DIRECTION ( 'NONE',  ( 2.603472992746261562E-14, 2.546204323184492723E-14, -1.000000000000000000 ) ) ;
#56075=AXIS2_PLACEMENT_3D ( 'NONE', #24594, #23132, #69716 ) ;
#56086=LINE ( 'NONE', #21873, #54973 ) ;
#56218=CARTESIAN_POINT ( 'NONE',  ( -2.410829926157000802E-12, -120.0000000000000000, 127.5000000000000000 ) ) ;
#56362=PLANE ( 'NONE',  #69353 ) ;
#56404=SURFACE_STYLE_FILL_AREA ( #57509 ) ;
#56411=CARTESIAN_POINT ( 'NONE',  ( 1.692257445284848207E-12, 0.000000000000000000, -65.00000000000000000 ) ) ;
#56483=PLANE ( 'NONE',  #47754 ) ;
#56506=VERTEX_POINT ( 'NONE', #57762 ) ;
#56592=CARTESIAN_POINT ( 'NONE',  ( -92.35000000002618492, -210.0000000000000853, -64.99999999999342037 ) ) ;
#56643=DIRECTION ( 'NONE',  ( -1.000000000000000000, 5.236901059551556403E-15, 2.618450529775778123E-14 ) ) ;
#56775=DIRECTION ( 'NONE',  ( 2.603472992746261562E-14, 2.546204323184492723E-14, -1.000000000000000000 ) ) ;
#56847=FACE_OUTER_BOUND ( 'NONE', #73144, .T. ) ;
#56861=VECTOR ( 'NONE', #70307, 1000.000000000000000 ) ;
#56864=ADVANCED_FACE ( 'NONE', ( #15864 ), #9849, .F. ) ;
#56931=CARTESIAN_POINT ( 'NONE',  ( -100.0000000000260485, 95.00000000000001421, 75.00000000000001421 ) ) ;
#57013=ORIENTED_EDGE ( 'NONE', *, *, #59794, .T. ) ;
#57149=ORIENTED_EDGE ( 'NONE', *, *, #71955, .T. ) ;
#57277=FACE_BOUND ( 'NONE', #8346, .T. ) ;
#57411=ORIENTED_EDGE ( 'NONE', *, *, #44071, .F. ) ;
#57509=FILL_AREA_STYLE ('',( #10514 ) ) ;
#57518=VERTEX_POINT ( 'NONE', #14484 ) ;
#57583=VECTOR ( 'NONE', #69826, 1000.000000000000000 ) ;
#57697=CARTESIAN_POINT ( 'NONE',  ( 12.75000000000024336, -120.0000000000000995, 127.4999999999996732 ) ) ;
#57762=CARTESIAN_POINT ( 'NONE',  ( 97.65000000002595471, -210.0000000000000853, -74.99999999999342037 ) ) ;
#57791=ADVANCED_FACE ( 'NONE', ( #12175 ), #46775, .F. ) ;
#57856=DIRECTION ( 'NONE',  ( 2.603472992746261562E-14, 2.546204323184492723E-14, -1.000000000000000000 ) ) ;
#57893=FACE_OUTER_BOUND ( 'NONE', #29055, .T. ) ;
#57952=DIRECTION ( 'NONE',  ( -1.000000000000000000, 7.955419762439749020E-15, 2.563413034563919251E-14 ) ) ;
#57957=CARTESIAN_POINT ( 'NONE',  ( 12.75000000000274447, -119.9999999999951257, -70.59999999999966747 ) ) ;
#58026=PRODUCT_DEFINITION_FORMATION_WITH_SPECIFIED_SOURCE ( 'ANY', '', #59551, .NOT_KNOWN. ) ;
#58103=VERTEX_POINT ( 'NONE', #58975 ) ;
#58123=DIRECTION ( 'NONE',  ( 2.603472992746261562E-14, 2.546204323184492723E-14, -1.000000000000000000 ) ) ;
#58147=EDGE_LOOP ( 'NONE', ( #9980, #11448 ) ) ;
#58248=EDGE_LOOP ( 'NONE', ( #38091, #46988 ) ) ;
#58557=CARTESIAN_POINT ( 'NONE',  ( -97.65000000002666525, 90.00000000000008527, -74.99999999999992895 ) ) ;
#58599=ORIENTED_EDGE ( 'NONE', *, *, #70861, .F. ) ;
#58688=CARTESIAN_POINT ( 'NONE',  ( 2.861260715122138586E-12, -120.0000000000000000, -75.00000000000000000 ) ) ;
#58691=CARTESIAN_POINT ( 'NONE',  ( 2.184357737007946383E-12, -120.0000000000000000, -48.99999999999997158 ) ) ;
#58712=EDGE_CURVE ( 'NONE', #18161, #21517, #61132, .T. ) ;
#58714=CARTESIAN_POINT ( 'NONE',  ( 97.65000000002652314, 90.00000000000005684, -75.00000000000007105 ) ) ;
#58728=EDGE_LOOP ( 'NONE', ( #57411, #4203, #18972, #59919 ) ) ;
#58915=( NAMED_UNIT ( * ) SI_UNIT ( $, .STERADIAN. ) SOLID_ANGLE_UNIT ( ) );
#58940=ORIENTED_EDGE ( 'NONE', *, *, #23292, .T. ) ;
#58975=CARTESIAN_POINT ( 'NONE',  ( -15.70000000000052687, -119.9999999999998721, -70.59999999999959641 ) ) ;
#58986=DIRECTION ( 'NONE',  ( 1.000000000000000000, -7.331661483372147883E-15, -2.592266024478009537E-14 ) ) ;
#59067=DIRECTION ( 'NONE',  ( 2.603472992746261562E-14, 2.546204323184492723E-14, -1.000000000000000000 ) ) ;
#59102=VERTEX_POINT ( 'NONE', #33566 ) ;
#59124=DIRECTION ( 'NONE',  ( 2.603472992745699578E-14, -2.546204323184531851E-14, 1.000000000000000000 ) ) ;
#59135=DIRECTION ( 'NONE',  ( -1.000000000000000000, 5.236901059551556403E-15, 2.618450529775778123E-14 ) ) ;
#59143=CARTESIAN_POINT ( 'NONE',  ( 2.600913415846943225E-12, -120.0000000000000000, -65.00000000000000000 ) ) ;
#59212=DIRECTION ( 'NONE',  ( -2.603472992746261562E-14, -2.546204323184492723E-14, 1.000000000000000000 ) ) ;
#59256=AXIS2_PLACEMENT_3D ( 'NONE', #15324, #9698, #27345 ) ;
#59259=DIRECTION ( 'NONE',  ( 2.603472992746261562E-14, 2.546204323184492723E-14, -1.000000000000000000 ) ) ;
#59394=AXIS2_PLACEMENT_3D ( 'NONE', #22553, #56775, #56015 ) ;
#59399=ORIENTED_EDGE ( 'NONE', *, *, #72073, .F. ) ;
#59551=PRODUCT ( 'housing cover', 'housing cover', '', ( #28664 ) ) ;
#59711=FACE_OUTER_BOUND ( 'NONE', #70580, .T. ) ;
#59760=CIRCLE ( 'NONE', #23735, 26.50000000000552092 ) ;
#59794=EDGE_CURVE ( 'NONE', #54110, #25904, #1879, .T. ) ;
#59888=DIRECTION ( 'NONE',  ( 2.603472992746261562E-14, 2.546204323184492723E-14, -1.000000000000000000 ) ) ;
#59919=ORIENTED_EDGE ( 'NONE', *, *, #31378, .F. ) ;
#59961=ORIENTED_EDGE ( 'NONE', *, *, #27260, .F. ) ;
#60264=AXIS2_PLACEMENT_3D ( 'NONE', #40261, #28976, #63210 ) ;
#60386=APPLICATION_CONTEXT ( 'automotive_design' ) ;
#60446=EDGE_CURVE ( 'NONE', #44982, #14031, #31938, .T. ) ;
#60584=EDGE_CURVE ( 'NONE', #25904, #14031, #28683, .T. ) ;
#60663=DIRECTION ( 'NONE',  ( -1.000000000000000000, 5.236901059551556403E-15, 2.618450529775778123E-14 ) ) ;
#60868=ORIENTED_EDGE ( 'NONE', *, *, #44237, .F. ) ;
#60965=DIRECTION ( 'NONE',  ( 1.000000000000000000, -1.047380211910311281E-14, -2.618450529775778123E-14 ) ) ;
#61040=CIRCLE ( 'NONE', #4609, 15.70000000000326956 ) ;
#61055=DIRECTION ( 'NONE',  ( 1.000000000000000000, -7.331661483372147883E-15, -2.618450529775767079E-14 ) ) ;
#61076=DIRECTION ( 'NONE',  ( 2.603472992746261562E-14, 2.546204323184492723E-14, -1.000000000000000000 ) ) ;
#61132=LINE ( 'NONE', #62630, #66738 ) ;
#61285=CARTESIAN_POINT ( 'NONE',  ( -23.50000000000271427, -119.9999999999998153, -48.99999999999936051 ) ) ;
#61304=EDGE_LOOP ( 'NONE', ( #56047, #46691 ) ) ;
#61350=DIRECTION ( 'NONE',  ( 2.603472992746261562E-14, 2.546204323184492723E-14, -1.000000000000000000 ) ) ;
#61486=CIRCLE ( 'NONE', #63862, 23.50000000000489919 ) ;
#61598=ORIENTED_EDGE ( 'NONE', *, *, #8050, .T. ) ;
#61606=DIRECTION ( 'NONE',  ( -1.000000000000000000, 1.047380211910311281E-14, 2.618450529775778123E-14 ) ) ;
#61695=VERTEX_POINT ( 'NONE', #51822 ) ;
#61770=ORIENTED_EDGE ( 'NONE', *, *, #42945, .T. ) ;
#61820=PLANE ( 'NONE',  #44738 ) ;
#61847=CARTESIAN_POINT ( 'NONE',  ( -0.0004442498507136653329, 0.001194404164628348752, -70.59999999999999432 ) ) ;
#61848=EDGE_LOOP ( 'NONE', ( #65698, #30337, #8892, #53578 ) ) ;
#61938=CARTESIAN_POINT ( 'NONE',  ( -26.49999999999739941, -119.9999999999996021, -65.00000000000069633 ) ) ;
#61946=CYLINDRICAL_SURFACE ( 'NONE', #69272, 26.50000000000552092 ) ;
#62046=ADVANCED_FACE ( 'NONE', ( #18031, #57893 ), #47703, .T. ) ;
#62087=LINE ( 'NONE', #33117, #24862 ) ;
#62241=ORIENTED_EDGE ( 'NONE', *, *, #38258, .T. ) ;
#62299=CARTESIAN_POINT ( 'NONE',  ( 2.184357737007946383E-12, -120.0000000000000000, -48.99999999999997158 ) ) ;
#62344=AXIS2_PLACEMENT_3D ( 'NONE', #17991, #57856, #34919 ) ;
#62386=DIRECTION ( 'NONE',  ( -7.616308197390131428E-15, 1.000000000000000000, -2.546204323184492723E-14 ) ) ;
#62402=EDGE_CURVE ( 'NONE', #63726, #29541, #5573, .T. ) ;
#62426=ORIENTED_EDGE ( 'NONE', *, *, #36743, .T. ) ;
#62430=ORIENTED_EDGE ( 'NONE', *, *, #50226, .T. ) ;
#62552=VERTEX_POINT ( 'NONE', #690 ) ;
#62630=CARTESIAN_POINT ( 'NONE',  ( -26.50044424985679825, 0.001194404164828994459, -48.99999999999931788 ) ) ;
#62724=DIRECTION ( 'NONE',  ( 2.603472992746261562E-14, 2.546204323184492723E-14, -1.000000000000000000 ) ) ;
#62733=EDGE_LOOP ( 'NONE', ( #57013, #62241 ) ) ;
#62782=FACE_OUTER_BOUND ( 'NONE', #47082, .T. ) ;
#62814=ORIENTED_EDGE ( 'NONE', *, *, #36743, .F. ) ;
#62826=ORIENTED_EDGE ( 'NONE', *, *, #21821, .T. ) ;
#62945=DIRECTION ( 'NONE',  ( 1.000000000000000000, -7.571541139944063212E-15, -2.603472992745718826E-14 ) ) ;
#63037=DIRECTION ( 'NONE',  ( 2.603472992746261562E-14, 2.546204323184492723E-14, -1.000000000000000000 ) ) ;
#63210=DIRECTION ( 'NONE',  ( -1.000000000000000000, 1.047380211910311281E-14, 2.618450529775778123E-14 ) ) ;
#63227=DIRECTION ( 'NONE',  ( 1.000000000000000000, -7.571539615859142926E-15, -2.618450529775767079E-14 ) ) ;
#63228=CIRCLE ( 'NONE', #17597, 26.50000000000552092 ) ;
#63291=CARTESIAN_POINT ( 'NONE',  ( 26.50000000000770939, -120.0000000000001847, -49.00000000000066080 ) ) ;
#63430=AXIS2_PLACEMENT_3D ( 'NONE', #74058, #22955, #50758 ) ;
#63442=EDGE_CURVE ( 'NONE', #43013, #64475, #531, .T. ) ;
#63489=VERTEX_POINT ( 'NONE', #41813 ) ;
#63565=CARTESIAN_POINT ( 'NONE',  ( 100.0000000000260343, -214.9999999999999716, 75.00000000000001421 ) ) ;
#63598=AXIS2_PLACEMENT_3D ( 'NONE', #49471, #32907, #15262 ) ;
#63658=VERTEX_POINT ( 'NONE', #50780 ) ;
#63681=DIRECTION ( 'NONE',  ( 2.603472992745699578E-14, -2.546204323184531851E-14, 1.000000000000000000 ) ) ;
#63726=VERTEX_POINT ( 'NONE', #29325 ) ;
#63862=AXIS2_PLACEMENT_3D ( 'NONE', #29334, #820, #34612 ) ;
#63910=ADVANCED_FACE ( 'NONE', ( #30434 ), #65050, .F. ) ;
#64046=DIRECTION ( 'NONE',  ( 1.000000000000000000, -7.571541139944063212E-15, -2.603472992745718826E-14 ) ) ;
#64179=EDGE_CURVE ( 'NONE', #27633, #17145, #25042, .T. ) ;
#64217=DIRECTION ( 'NONE',  ( 1.000000000000000000, -7.571537405616606460E-15, -2.598394312951952234E-14 ) ) ;
#64220=EDGE_LOOP ( 'NONE', ( #49909, #47930 ) ) ;
#64267=ORIENTED_EDGE ( 'NONE', *, *, #42054, .F. ) ;
#64363=DIRECTION ( 'NONE',  ( 2.603472992746261562E-14, 2.546204323184492723E-14, -1.000000000000000000 ) ) ;
#64388=CIRCLE ( 'NONE', #69217, 2.650000000000540812 ) ;
#64459=EDGE_LOOP ( 'NONE', ( #5225, #30765, #6748, #54856 ) ) ;
#64475=VERTEX_POINT ( 'NONE', #15550 ) ;
#64516=DIRECTION ( 'NONE',  ( 2.603472992746261562E-14, 2.546204323184492723E-14, -1.000000000000000000 ) ) ;
#64566=ORIENTED_EDGE ( 'NONE', *, *, #64179, .T. ) ;
#64592=LINE ( 'NONE', #71318, #12841 ) ;
#64620=VERTEX_POINT ( 'NONE', #73791 ) ;
#64865=AXIS2_PLACEMENT_3D ( 'NONE', #5966, #67613, #61606 ) ;
#64926=EDGE_CURVE ( 'NONE', #32262, #63489, #38019, .T. ) ;
#65050=CYLINDRICAL_SURFACE ( 'NONE', #35953, 2.650000000000540812 ) ;
#65276=FILL_AREA_STYLE_COLOUR ( '', #5079 ) ;
#65517=DIRECTION ( 'NONE',  ( -2.603472992746261562E-14, -2.546204323184492723E-14, 1.000000000000000000 ) ) ;
#65608=CARTESIAN_POINT ( 'NONE',  ( -100.0000000000260059, -214.9999999999999716, -64.99999999999350564 ) ) ;
#65698=ORIENTED_EDGE ( 'NONE', *, *, #66954, .F. ) ;
#65731=FACE_OUTER_BOUND ( 'NONE', #26133, .T. ) ;
#65815=CIRCLE ( 'NONE', #55010, 2.650000000000540812 ) ;
#65821=DIRECTION ( 'NONE',  ( 2.603472992746261562E-14, 2.546204323184492723E-14, -1.000000000000000000 ) ) ;
#65908=AXIS2_PLACEMENT_3D ( 'NONE', #56411, #16541, #38365 ) ;
#66075=FACE_OUTER_BOUND ( 'NONE', #50295, .T. ) ;
#66193=AXIS2_PLACEMENT_3D ( 'NONE', #30181, #63681, #64046 ) ;
#66229=DIRECTION ( 'NONE',  ( -1.000000000000000000, 7.571537405616606460E-15, 2.598394312951952234E-14 ) ) ;
#66412=DIRECTION ( 'NONE',  ( 1.000000000000000000, -1.047380211910311281E-14, -2.618450529775778123E-14 ) ) ;
#66416=ORIENTED_EDGE ( 'NONE', *, *, #48450, .F. ) ;
#66485=EDGE_LOOP ( 'NONE', ( #26638, #28275, #11616, #34280 ) ) ;
#66507=ORIENTED_EDGE ( 'NONE', *, *, #45923, .T. ) ;
#66530=CYLINDRICAL_SURFACE ( 'NONE', #43360, 2.650000000000540812 ) ;
#66719=CYLINDRICAL_SURFACE ( 'NONE', #18739, 15.70000000000327312 ) ;
#66738=VECTOR ( 'NONE', #11106, 1000.000000000000000 ) ;
#66777=VECTOR ( 'NONE', #69656, 1000.000000000000000 ) ;
#66779=DIRECTION ( 'NONE',  ( 1.000000000000000000, -7.331661483372147883E-15, -2.592266024478009537E-14 ) ) ;
#66812=CARTESIAN_POINT ( 'NONE',  ( 100.0000000000260343, -214.9999999999999716, -74.99999999999349143 ) ) ;
#66814=LINE ( 'NONE', #31846, #54586 ) ;
#66841=CYLINDRICAL_SURFACE ( 'NONE', #59256, 15.70000000000327312 ) ;
#66851=EDGE_LOOP ( 'NONE', ( #36965, #12199, #27535, #72501 ) ) ;
#66896=DIRECTION ( 'NONE',  ( 2.603472992746261562E-14, 2.546204323184492723E-14, -1.000000000000000000 ) ) ;
#66954=EDGE_CURVE ( 'NONE', #73822, #30711, #39441, .T. ) ;
#66980=AXIS2_PLACEMENT_3D ( 'NONE', #41691, #30402, #46237 ) ;
#66995=DIRECTION ( 'NONE',  ( -1.000000000000000000, 7.571543891232750625E-15, 2.563413034563919882E-14 ) ) ;
#67107=VERTEX_POINT ( 'NONE', #69844 ) ;
#67116=VECTOR ( 'NONE', #14296, 1000.000000000000000 ) ;
#67135=SHAPE_REPRESENTATION ( 'housing cover', ( #43395 ), #37485 ) ;
#67136=CARTESIAN_POINT ( 'NONE',  ( -97.65000000002666525, 90.00000000000008527, -74.99999999999992895 ) ) ;
#67148=EDGE_CURVE ( 'NONE', #27140, #57518, #21002, .T. ) ;
#67179=DIRECTION ( 'NONE',  ( 2.603472992746261562E-14, 2.546204323184492723E-14, -1.000000000000000000 ) ) ;
#67288=DIRECTION ( 'NONE',  ( 2.603472992746261562E-14, 2.546204323184492723E-14, -1.000000000000000000 ) ) ;
#67448=FACE_BOUND ( 'NONE', #64220, .T. ) ;
#67455=DIRECTION ( 'NONE',  ( 1.000000000000000000, -7.571539615859142926E-15, -2.618450529775767079E-14 ) ) ;
#67476=EDGE_CURVE ( 'NONE', #18206, #58103, #46299, .T. ) ;
#67517=EDGE_LOOP ( 'NONE', ( #47994, #58940 ) ) ;
#67613=DIRECTION ( 'NONE',  ( 2.603472992746261562E-14, 2.546204323184492723E-14, -1.000000000000000000 ) ) ;
#67637=FACE_OUTER_BOUND ( 'NONE', #7863, .T. ) ;
#67682=PLANE ( 'NONE',  #65908 ) ;
#67912=CARTESIAN_POINT ( 'NONE',  ( 95.00000000002597744, 90.00000000000007105, -75.00000000000000000 ) ) ;
#67933=ADVANCED_FACE ( 'NONE', ( #43802 ), #66719, .F. ) ;
#67968=EDGE_CURVE ( 'NONE', #21517, #29541, #46348, .T. ) ;
#67969=AXIS2_PLACEMENT_3D ( 'NONE', #56931, #8272, #32301 ) ;
#67984=DIRECTION ( 'NONE',  ( 2.603472992746261562E-14, 2.546204323184492723E-14, -1.000000000000000000 ) ) ;
#68005=FACE_BOUND ( 'NONE', #29215, .T. ) ;
#68008=UNCERTAINTY_MEASURE_WITH_UNIT (LENGTH_MEASURE( 1.000000000000000082E-05 ), #46513, 'distance_accuracy_value', 'NONE');
#68101=ADVANCED_FACE ( 'NONE', ( #48135 ), #16699, .F. ) ;
#68174=VECTOR ( 'NONE', #62724, 1000.000000000000000 ) ;
#68252=ORIENTED_EDGE ( 'NONE', *, *, #53661, .F. ) ;
#68263=ORIENTED_EDGE ( 'NONE', *, *, #58712, .T. ) ;
#68414=ORIENTED_EDGE ( 'NONE', *, *, #45524, .F. ) ;
#68669=CARTESIAN_POINT ( 'NONE',  ( 2.746707903440850533E-12, -120.0000000000000000, -70.59999999999999432 ) ) ;
#68715=( GEOMETRIC_REPRESENTATION_CONTEXT ( 3 ) GLOBAL_UNCERTAINTY_ASSIGNED_CONTEXT ( ( #68008 ) ) GLOBAL_UNIT_ASSIGNED_CONTEXT ( ( #46513, #69804, #58915 ) ) REPRESENTATION_CONTEXT ( 'NONE', 'WORKASPACE' ) );
#68759=DIRECTION ( 'NONE',  ( -1.000000000000000000, 7.571544473058805744E-15, 2.612289469705706870E-14 ) ) ;
#68984=AXIS2_PLACEMENT_3D ( 'NONE', #69234, #28628, #6460 ) ;
#69047=CIRCLE ( 'NONE', #51006, 12.75000000000265565 ) ;
#69127=EDGE_LOOP ( 'NONE', ( #149, #59399 ) ) ;
#69137=CYLINDRICAL_SURFACE ( 'NONE', #26791, 2.650000000000540812 ) ;
#69152=DIRECTION ( 'NONE',  ( -1.000000000000000000, 7.619177619974977057E-15, 2.612289469705706555E-14 ) ) ;
#69217=AXIS2_PLACEMENT_3D ( 'NONE', #42578, #65517, #13989 ) ;
#69234=CARTESIAN_POINT ( 'NONE',  ( 95.00000000002596323, -209.9999999999999147, -74.99999999999349143 ) ) ;
#69272=AXIS2_PLACEMENT_3D ( 'NONE', #50649, #45407, #10430 ) ;
#69353=AXIS2_PLACEMENT_3D ( 'NONE', #5609, #41551, #16499 ) ;
#69498=DIRECTION ( 'NONE',  ( -1.000000000000000000, 7.571544473058805744E-15, 2.612289469705706870E-14 ) ) ;
#69582=ORIENTED_EDGE ( 'NONE', *, *, #59794, .F. ) ;
#69605=EDGE_CURVE ( 'NONE', #57518, #27140, #18954, .T. ) ;
#69656=DIRECTION ( 'NONE',  ( 2.603472992746261562E-14, 2.546204323184492723E-14, -1.000000000000000000 ) ) ;
#69716=DIRECTION ( 'NONE',  ( -1.000000000000000000, 7.571539615859142926E-15, 2.592266024478009537E-14 ) ) ;
#69804=( NAMED_UNIT ( * ) PLANE_ANGLE_UNIT ( ) SI_UNIT ( $, .RADIAN. ) );
#69812=EDGE_CURVE ( 'NONE', #63658, #15051, #56086, .T. ) ;
#69826=DIRECTION ( 'NONE',  ( -7.616308197390131428E-15, 1.000000000000000000, -2.546204323184492723E-14 ) ) ;
#69844=CARTESIAN_POINT ( 'NONE',  ( -23.50044424985128089, 0.001194404165009976208, -49.00000000000061107 ) ) ;
#69910=EDGE_CURVE ( 'NONE', #29541, #21517, #59760, .T. ) ;
#70051=VECTOR ( 'NONE', #67179, 1000.000000000000000 ) ;
#70091=CARTESIAN_POINT ( 'NONE',  ( -100.0000000000260485, 95.00000000000001421, -65.00000000000001421 ) ) ;
#70144=ORIENTED_EDGE ( 'NONE', *, *, #7414, .F. ) ;
#70189=ORIENTED_EDGE ( 'NONE', *, *, #235, .F. ) ;
#70261=ORIENTED_EDGE ( 'NONE', *, *, #60446, .F. ) ;
#70284=EDGE_CURVE ( 'NONE', #42522, #61695, #32409, .T. ) ;
#70307=DIRECTION ( 'NONE',  ( 2.603472992746261562E-14, 2.546204323184492723E-14, -1.000000000000000000 ) ) ;
#70318=EDGE_CURVE ( 'NONE', #15051, #30682, #61040, .T. ) ;
#70321=ORIENTED_EDGE ( 'NONE', *, *, #62402, .T. ) ;
#70374=CARTESIAN_POINT ( 'NONE',  ( -12.75044424985336633, 0.001194404164724885897, -70.59999999999966747 ) ) ;
#70392=DIRECTION ( 'NONE',  ( -1.000000000000000000, 1.047380211910311281E-14, 2.618450529775778123E-14 ) ) ;
#70534=CARTESIAN_POINT ( 'NONE',  ( -95.00000000002617639, -209.9999999999999432, -64.99999999999349143 ) ) ;
#70535=AXIS2_PLACEMENT_3D ( 'NONE', #59143, #24920, #19641 ) ;
#70540=ORIENTED_EDGE ( 'NONE', *, *, #64926, .T. ) ;
#70571=LINE ( 'NONE', #13451, #4973 ) ;
#70580=EDGE_LOOP ( 'NONE', ( #12972, #40682, #62426, #19004 ) ) ;
#70585=EDGE_CURVE ( 'NONE', #40286, #50011, #28670, .T. ) ;
#70641=CARTESIAN_POINT ( 'NONE',  ( -100.0000000000260485, 95.00000000000001421, 75.00000000000001421 ) ) ;
#70688=VECTOR ( 'NONE', #28965, 1000.000000000000000 ) ;
#70790=CIRCLE ( 'NONE', #47995, 23.50000000000489919 ) ;
#70861=EDGE_CURVE ( 'NONE', #53187, #59102, #4524, .T. ) ;
#70951=CARTESIAN_POINT ( 'NONE',  ( -15.70000000000041140, -119.9999999999998721, -74.99999999999958789 ) ) ;
#70970=CARTESIAN_POINT ( 'NONE',  ( -97.65000000002611102, 89.99999999999995737, -65.00000000000007105 ) ) ;
#71116=FACE_BOUND ( 'NONE', #14235, .T. ) ;
#71142=DIRECTION ( 'NONE',  ( 1.000000000000000000, -7.571541139944063212E-15, -2.603472992745718510E-14 ) ) ;
#71232=DIRECTION ( 'NONE',  ( 0.000000000000000000, 0.000000000000000000, 1.000000000000000000 ) ) ;
#71318=CARTESIAN_POINT ( 'NONE',  ( 12.74955575014678288, 0.001194404164533373076, 127.4927882439599927 ) ) ;
#71462=EDGE_LOOP ( 'NONE', ( #35420, #61770 ) ) ;
#71503=VECTOR ( 'NONE', #73446, 1000.000000000000000 ) ;
#71520=EDGE_CURVE ( 'NONE', #30711, #61695, #51759, .T. ) ;
#71589=DIRECTION ( 'NONE',  ( 2.603472992746261562E-14, 2.546204323184492723E-14, -1.000000000000000000 ) ) ;
#71592=LINE ( 'NONE', #65608, #21692 ) ;
#71599=DIRECTION ( 'NONE',  ( 1.000000000000000000, -5.236901059551556403E-15, -2.618450529775778123E-14 ) ) ;
#71627=ORIENTED_EDGE ( 'NONE', *, *, #67476, .T. ) ;
#71644=ORIENTED_EDGE ( 'NONE', *, *, #24639, .T. ) ;
#71771=DIRECTION ( 'NONE',  ( 2.603472992746261562E-14, 2.546204323184492723E-14, -1.000000000000000000 ) ) ;
#71955=EDGE_CURVE ( 'NONE', #46060, #29601, #10809, .T. ) ;
#72047=AXIS2_PLACEMENT_3D ( 'NONE', #25645, #36924, #60965 ) ;
#72050=ADVANCED_FACE ( 'NONE', ( #33382 ), #34504, .F. ) ;
#72073=EDGE_CURVE ( 'NONE', #56506, #64475, #22839, .T. ) ;
#72149=AXIS2_PLACEMENT_3D ( 'NONE', #70641, #53013, #42105 ) ;
#72345=EDGE_LOOP ( 'NONE', ( #36969, #41500, #18416, #47727 ) ) ;
#72482=EDGE_CURVE ( 'NONE', #50011, #40286, #51702, .T. ) ;
#72501=ORIENTED_EDGE ( 'NONE', *, *, #46112, .F. ) ;
#72569=ORIENTED_EDGE ( 'NONE', *, *, #23448, .T. ) ;
#72610=CARTESIAN_POINT ( 'NONE',  ( 2.184357737007946383E-12, -120.0000000000000000, -48.99999999999997158 ) ) ;
#72948=EDGE_CURVE ( 'NONE', #53187, #62552, #70790, .T. ) ;
#73077=CARTESIAN_POINT ( 'NONE',  ( -0.0004442498508594591917, 0.001194404164628348752, -65.00000000000000000 ) ) ;
#73106=AXIS2_PLACEMENT_3D ( 'NONE', #22230, #61350, #55700 ) ;
#73144=EDGE_LOOP ( 'NONE', ( #5837, #7840, #18492, #41878 ) ) ;
#73241=CARTESIAN_POINT ( 'NONE',  ( -0.0004442498558709490585, 0.001194404164628348752, 127.4927882439603195 ) ) ;
#73441=ORIENTED_EDGE ( 'NONE', *, *, #44071, .T. ) ;
#73446=DIRECTION ( 'NONE',  ( 2.603472992746261562E-14, 2.546204323184492723E-14, -1.000000000000000000 ) ) ;
#73641=AXIS2_PLACEMENT_3D ( 'NONE', #17908, #17537, #46481 ) ;
#73689=CIRCLE ( 'NONE', #20885, 23.50000000000489919 ) ;
#73791=CARTESIAN_POINT ( 'NONE',  ( 92.35000000002600018, 89.99999999999995737, -65.00000000000007105 ) ) ;
#73811=ORIENTED_EDGE ( 'NONE', *, *, #6400, .T. ) ;
#73817=CIRCLE ( 'NONE', #54614, 2.650000000000540812 ) ;
#73822=VERTEX_POINT ( 'NONE', #66812 ) ;
#73851=DIRECTION ( 'NONE',  ( 2.603472992746261562E-14, 2.546204323184492723E-14, -1.000000000000000000 ) ) ;
#73895=CARTESIAN_POINT ( 'NONE',  ( -100.0000000000260059, -214.9999999999999716, -74.99999999999349143 ) ) ;
#73975=ORIENTED_EDGE ( 'NONE', *, *, #72948, .F. ) ;
#74058=CARTESIAN_POINT ( 'NONE',  ( -0.0004442498507136653329, 0.001194404164628348752, -70.59999999999999432 ) ) ;
#74179=DIRECTION ( 'NONE',  ( -2.603472992746261562E-14, -2.546204323184492723E-14, 1.000000000000000000 ) ) ;
#74197=DIRECTION ( 'NONE',  ( 2.603472992746261562E-14, 2.546204323184492723E-14, -1.000000000000000000 ) ) ;
#74243=VECTOR ( 'NONE', #11423, 1000.000000000000000 ) ;
#74300=AXIS2_PLACEMENT_3D ( 'NONE', #58688, #59067, #57952 ) ;
#74305=CARTESIAN_POINT ( 'NONE',  ( 12.75000000000259881, -119.9999999999951257, -64.99999999999967315 ) ) ;
#74330=FACE_OUTER_BOUND ( 'NONE', #18635, .T. ) ;
ENDSEC;
END-ISO-10303-21;
